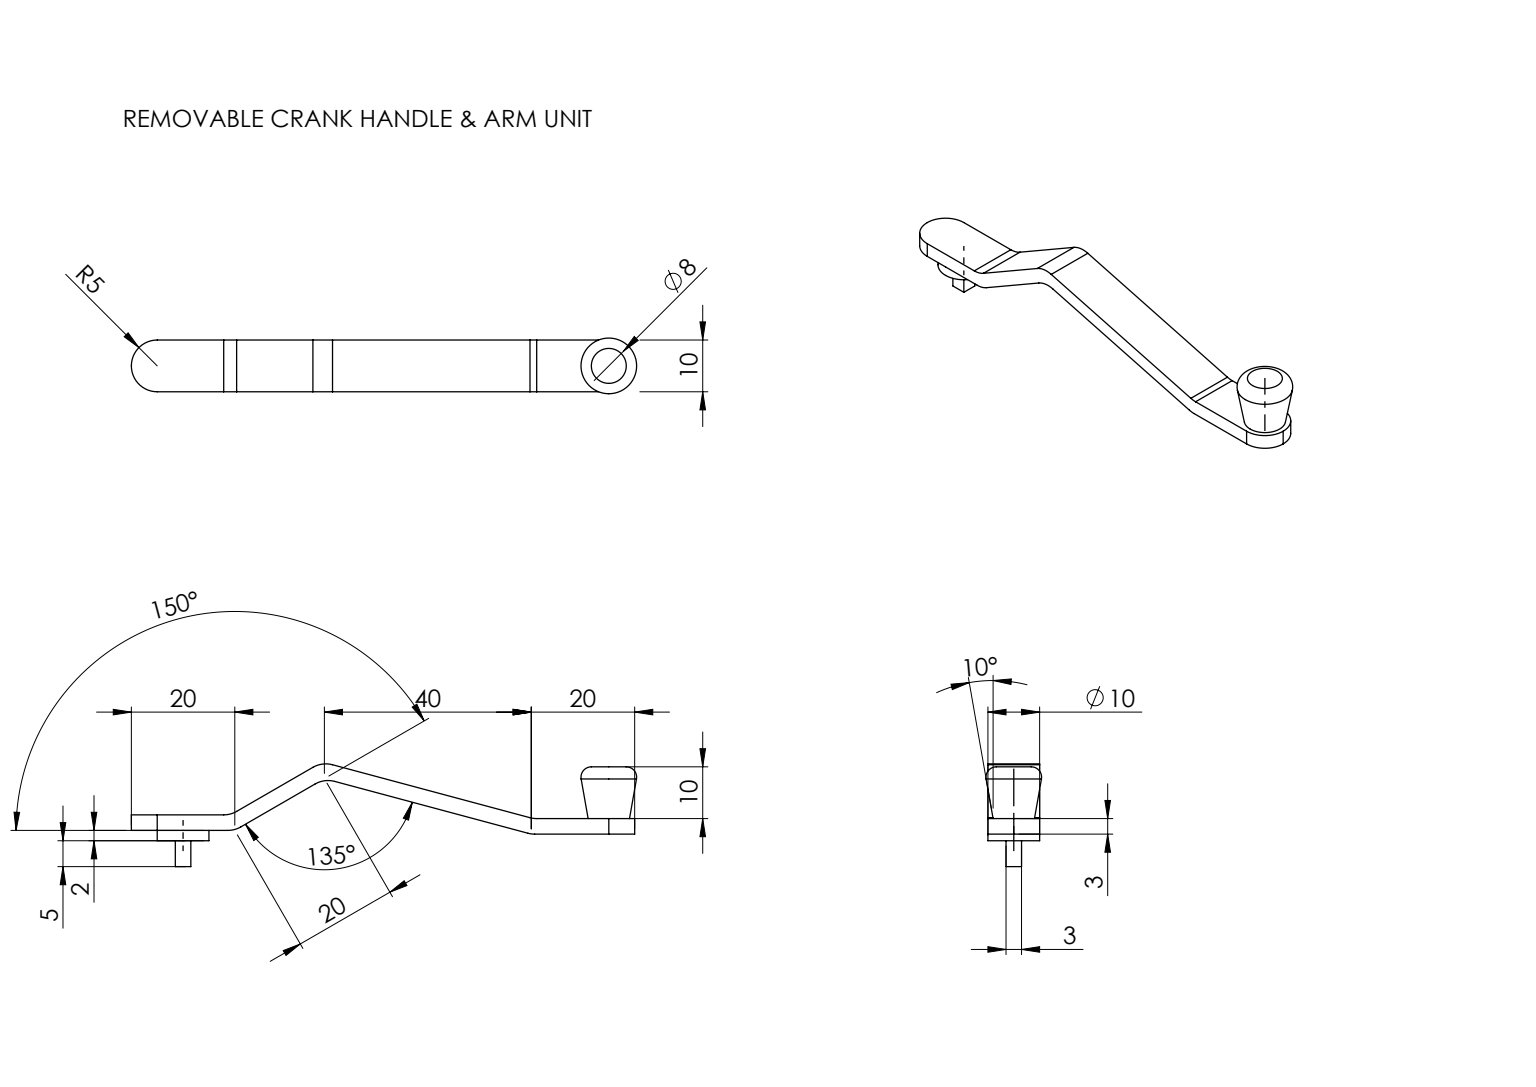
ISO-10303-21;
HEADER;
FILE_DESCRIPTION (('STEP AP214'),
    '1' );
FILE_NAME ('Removable Crank Handle & Arm Unit.step',
    '2026-10-04T07:23:31',
    ( '' ),
    ( '' ),
    'SwSTEP 2.0',
    'SolidWorks 2026',
    '' );
FILE_SCHEMA (( 'AUTOMOTIVE_DESIGN' ));
ENDSEC;

DATA;
#3=ORIENTED_EDGE ( 'NONE', *, *, #5333, .F. ) ;
#12=CARTESIAN_POINT ( 'NONE',  ( 10.00000000000000000, 90.00000000000001421, -5.000000000000000000 ) ) ;
#31=VECTOR ( 'NONE', #278, 1000.000000000000000 ) ;
#33=ORIENTED_EDGE ( 'NONE', *, *, #3191, .T. ) ;
#67=ORIENTED_EDGE ( 'NONE', *, *, #4182, .T. ) ;
#77=ORIENTED_EDGE ( 'NONE', *, *, #7857, .F. ) ;
#83=ORIENTED_EDGE ( 'NONE', *, *, #9025, .F. ) ;
#91=CARTESIAN_POINT ( 'NONE',  ( 1.040834085586084257E-14, 88.00000000000001421, -4.999999999999987566 ) ) ;
#96=SURFACE_SIDE_STYLE ('',( #6842 ) ) ;
#100=LINE ( 'NONE', #5208, #8824 ) ;
#110=DIRECTION ( 'NONE',  ( 0.000000000000000000, 0.000000000000000000, 1.000000000000000000 ) ) ;
#142=ORIENTED_EDGE ( 'NONE', *, *, #10441, .F. ) ;
#177=ADVANCED_FACE ( 'NONE', ( #4290 ), #10361, .F. ) ;
#191=DIRECTION ( 'NONE',  ( 1.000000000000000000, 0.000000000000000000, 0.000000000000000000 ) ) ;
#194=FACE_OUTER_BOUND ( 'NONE', #6105, .T. ) ;
#206=EDGE_LOOP ( 'NONE', ( #9870, #5506, #9937, #2232 ) ) ;
#224=VECTOR ( 'NONE', #10052, 1000.000000000000000 ) ;
#227=CIRCLE ( 'NONE', #6760, 2.000000000000000000 ) ;
#242=ORIENTED_EDGE ( 'NONE', *, *, #1929, .F. ) ;
#243=CIRCLE ( 'NONE', #1136, 3.379762621896238883 ) ;
#250=EDGE_CURVE ( 'NONE', #1860, #1446, #9645, .T. ) ;
#257=VERTEX_POINT ( 'NONE', #2223 ) ;
#259=ORIENTED_EDGE ( 'NONE', *, *, #4096, .F. ) ;
#265=CARTESIAN_POINT ( 'NONE',  ( -1.500000000000000444, 88.00000000000001421, -1.500000000000000222 ) ) ;
#267=DIRECTION ( 'NONE',  ( 0.000000000000000000, 0.000000000000000000, -1.000000000000000000 ) ) ;
#268=EDGE_CURVE ( 'NONE', #2208, #3766, #1396, .T. ) ;
#278=DIRECTION ( 'NONE',  ( -0.000000000000000000, 1.000000000000000000, -0.000000000000000000 ) ) ;
#314=CARTESIAN_POINT ( 'NONE',  ( -5.000000000000000000, 90.00000000000001421, 0.000000000000000000 ) ) ;
#327=CARTESIAN_POINT ( 'NONE',  ( 82.32050807568876394, 92.28203230275514102, 5.000000000000000000 ) ) ;
#347=PRODUCT_DEFINITION_FORMATION_WITH_SPECIFIED_SOURCE ( 'ANY', '', #361, .NOT_KNOWN. ) ;
#361=PRODUCT ( 'Removable Crank Handle & Arm Unit', 'Removable Crank Handle & Arm Unit', '', ( #7853 ) ) ;
#365=DIRECTION ( 'NONE',  ( -0.000000000000000000, -1.000000000000000000, -0.000000000000000000 ) ) ;
#366=ORIENTED_EDGE ( 'NONE', *, *, #7588, .T. ) ;
#367=DIRECTION ( 'NONE',  ( -1.000000000000000000, 5.551115123125781913E-15, 0.000000000000000000 ) ) ;
#371=DIRECTION ( 'NONE',  ( 0.000000000000000000, -0.000000000000000000, 1.000000000000000000 ) ) ;
#377=EDGE_CURVE ( 'NONE', #6765, #3339, #3870, .T. ) ;
#381=DIRECTION ( 'NONE',  ( 0.000000000000000000, 0.000000000000000000, 1.000000000000000000 ) ) ;
#383=ORIENTED_EDGE ( 'NONE', *, *, #5717, .F. ) ;
#385=DIRECTION ( 'NONE',  ( -0.000000000000000000, 1.000000000000000000, -0.000000000000000000 ) ) ;
#387=VERTEX_POINT ( 'NONE', #2812 ) ;
#408=FILL_AREA_STYLE ('',( #5487 ) ) ;
#422=CARTESIAN_POINT ( 'NONE',  ( 1.499999999999999556, 83.00000000000000000, -1.500000000000000222 ) ) ;
#435=DIRECTION ( 'NONE',  ( 0.000000000000000000, 0.000000000000000000, 1.000000000000000000 ) ) ;
#440=LINE ( 'NONE', #3807, #6013 ) ;
#467=ADVANCED_FACE ( 'NONE', ( #4314 ), #3524, .F. ) ;
#470=CARTESIAN_POINT ( 'NONE',  ( -5.000000000000000000, 93.00000000000001421, 0.000000000000000000 ) ) ;
#490=CARTESIAN_POINT ( 'NONE',  ( 1.040834085586084257E-14, 90.00000000000001421, 5.000000000000000000 ) ) ;
#491=CARTESIAN_POINT ( 'NONE',  ( -1.500000000000000444, 88.00000000000001421, 1.499999999999999778 ) ) ;
#505=ORIENTED_EDGE ( 'NONE', *, *, #6617, .F. ) ;
#514=VERTEX_POINT ( 'NONE', #5086 ) ;
#521=CARTESIAN_POINT ( 'NONE',  ( -5.000000000000000000, 93.00000000000001421, 5.000000000000000000 ) ) ;
#529=DIRECTION ( 'NONE',  ( 0.000000000000000000, 0.000000000000000000, -1.000000000000000000 ) ) ;
#533=EDGE_CURVE ( 'NONE', #8829, #4450, #8962, .T. ) ;
#535=CARTESIAN_POINT ( 'NONE',  ( 1.040834085586084257E-14, 90.00000000000001421, 0.000000000000000000 ) ) ;
#544=VERTEX_POINT ( 'NONE', #8636 ) ;
#546=CARTESIAN_POINT ( 'NONE',  ( -1.500000000000000444, 83.00000000000000000, 1.499999999999999778 ) ) ;
#549=ORIENTED_EDGE ( 'NONE', *, *, #6741, .T. ) ;
#564=VERTEX_POINT ( 'NONE', #7642 ) ;
#574=EDGE_CURVE ( 'NONE', #8829, #3039, #9473, .T. ) ;
#587=AXIS2_PLACEMENT_3D ( 'NONE', #4145, #5850, #2623 ) ;
#590=DIRECTION ( 'NONE',  ( -1.000000000000000000, 0.000000000000000000, 0.000000000000000000 ) ) ;
#618=CARTESIAN_POINT ( 'NONE',  ( 8.660254037844401509, 90.00000000000001421, -5.000000000000000000 ) ) ;
#625=ORIENTED_EDGE ( 'NONE', *, *, #3191, .F. ) ;
#648=FACE_OUTER_BOUND ( 'NONE', #8082, .T. ) ;
#653=DIRECTION ( 'NONE',  ( 0.000000000000000000, -0.000000000000000000, 1.000000000000000000 ) ) ;
#658=EDGE_CURVE ( 'NONE', #10864, #2380, #8577, .T. ) ;
#663=CARTESIAN_POINT ( 'NONE',  ( 67.32050807568876394, 89.28203230275514102, 5.000000000000000000 ) ) ;
#672=CIRCLE ( 'NONE', #9503, 2.000000000000000000 ) ;
#677=ORIENTED_EDGE ( 'NONE', *, *, #2132, .T. ) ;
#706=LINE ( 'NONE', #4869, #4614 ) ;
#709=CARTESIAN_POINT ( 'NONE',  ( 67.07963283087528339, 92.45240317130979690, -5.000000000000000000 ) ) ;
#711=EDGE_CURVE ( 'NONE', #8862, #6537, #6673, .T. ) ;
#719=DIRECTION ( 'NONE',  ( -0.000000000000000000, -1.000000000000000000, -0.000000000000000000 ) ) ;
#725=FACE_OUTER_BOUND ( 'NONE', #3287, .T. ) ;
#754=DIRECTION ( 'NONE',  ( 0.000000000000000000, 1.000000000000000000, 0.000000000000000000 ) ) ;
#770=DIRECTION ( 'NONE',  ( 0.000000000000000000, 0.000000000000000000, -1.000000000000000000 ) ) ;
#782=LINE ( 'NONE', #4259, #4639 ) ;
#796=ORIENTED_EDGE ( 'NONE', *, *, #6662, .F. ) ;
#806=VERTEX_POINT ( 'NONE', #6323 ) ;
#810=EDGE_CURVE ( 'NONE', #5184, #1232, #9685, .T. ) ;
#821=FACE_OUTER_BOUND ( 'NONE', #5736, .T. ) ;
#828=DIRECTION ( 'NONE',  ( 0.000000000000000000, -0.000000000000000000, 1.000000000000000000 ) ) ;
#836=FACE_OUTER_BOUND ( 'NONE', #7251, .T. ) ;
#838=CARTESIAN_POINT ( 'NONE',  ( 7.856406460551036197, 93.00000000000001421, -5.000000000000000000 ) ) ;
#839=LINE ( 'NONE', #6642, #10047 ) ;
#862=FACE_OUTER_BOUND ( 'NONE', #9094, .T. ) ;
#875=ORIENTED_EDGE ( 'NONE', *, *, #1882, .T. ) ;
#878=CARTESIAN_POINT ( 'NONE',  ( 8.660254037844401509, 90.00000000000001421, 5.000000000000000000 ) ) ;
#885=VECTOR ( 'NONE', #3233, 1000.000000000000000 ) ;
#894=DIRECTION ( 'NONE',  ( 0.000000000000000000, -0.000000000000000000, 1.000000000000000000 ) ) ;
#898=AXIS2_PLACEMENT_3D ( 'NONE', #9603, #2840, #2892 ) ;
#922=DIRECTION ( 'NONE',  ( -1.000000000000000000, 0.000000000000000000, 0.000000000000000000 ) ) ;
#926=CONICAL_SURFACE ( 'NONE', #3744, 4.000000000000006217, 0.1745329251994333364 ) ;
#934=ORIENTED_EDGE ( 'NONE', *, *, #377, .T. ) ;
#937=CARTESIAN_POINT ( 'NONE',  ( 28.02691073765301155, 94.63433907514509258, 5.000000000000000000 ) ) ;
#944=DIRECTION ( 'NONE',  ( -0.000000000000000000, -0.000000000000000000, 1.000000000000000000 ) ) ;
#955=CARTESIAN_POINT ( 'NONE',  ( 28.89716436598705585, 102.6833647615033840, -5.000000000000000000 ) ) ;
#956=VERTEX_POINT ( 'NONE', #4935 ) ;
#973=FACE_OUTER_BOUND ( 'NONE', #9739, .T. ) ;
#977=ORIENTED_EDGE ( 'NONE', *, *, #1807, .T. ) ;
#1000=CARTESIAN_POINT ( 'NONE',  ( 1.500000000000000000, 83.00000000000000000, 1.500000000000000000 ) ) ;
#1002=ORIENTED_EDGE ( 'NONE', *, *, #1471, .T. ) ;
#1031=DIRECTION ( 'NONE',  ( 0.9659258262890684232, -0.2588190451025202399, 0.000000000000000000 ) ) ;
#1041=DIRECTION ( 'NONE',  ( 0.2588190451025202399, 0.9659258262890684232, -0.000000000000000000 ) ) ;
#1045=CARTESIAN_POINT ( 'NONE',  ( 0.000000000000000000, 83.00000000000000000, 0.000000000000000000 ) ) ;
#1047=AXIS2_PLACEMENT_3D ( 'NONE', #1899, #5280, #4212 ) ;
#1058=ADVANCED_FACE ( 'NONE', ( #4325 ), #4262, .T. ) ;
#1067=PLANE ( 'NONE',  #8873 ) ;
#1072=EDGE_LOOP ( 'NONE', ( #5589, #3090, #10487, #3502 ) ) ;
#1093=ORIENTED_EDGE ( 'NONE', *, *, #10175, .T. ) ;
#1115=CARTESIAN_POINT ( 'NONE',  ( -5.000000000000000000, 90.00000000000001421, 0.000000000000000000 ) ) ;
#1125=VECTOR ( 'NONE', #3487, 1000.000000000000000 ) ;
#1136=AXIS2_PLACEMENT_3D ( 'NONE', #9771, #8895, #5691 ) ;
#1143=ADVANCED_FACE ( 'NONE', ( #648 ), #10756, .F. ) ;
#1160=DIRECTION ( 'NONE',  ( 0.000000000000000000, 0.000000000000000000, 1.000000000000000000 ) ) ;
#1179=CARTESIAN_POINT ( 'NONE',  ( 67.07963283087528339, 92.45240317130979690, 5.000000000000000000 ) ) ;
#1192=DIRECTION ( 'NONE',  ( -0.8660254037844382635, -0.5000000000000004441, 0.000000000000000000 ) ) ;
#1211=EDGE_LOOP ( 'NONE', ( #2757, #9774 ) ) ;
#1216=EDGE_CURVE ( 'NONE', #2617, #9902, #2682, .T. ) ;
#1220=CARTESIAN_POINT ( 'NONE',  ( -1.500000000000000444, 83.00000000000000000, -1.500000000000000222 ) ) ;
#1232=VERTEX_POINT ( 'NONE', #9251 ) ;
#1240=LINE ( 'NONE', #4680, #1791 ) ;
#1249=CIRCLE ( 'NONE', #1405, 5.000000000000000888 ) ;
#1251=DIRECTION ( 'NONE',  ( -0.000000000000000000, -0.000000000000000000, 1.000000000000000000 ) ) ;
#1261=AXIS2_PLACEMENT_3D ( 'NONE', #3295, #5864, #9221 ) ;
#1268=CARTESIAN_POINT ( 'NONE',  ( 28.89716436598705585, 102.6833647615033840, 5.000000000000000000 ) ) ;
#1272=CIRCLE ( 'NONE', #4980, 5.000000000000000000 ) ;
#1281=DIRECTION ( 'NONE',  ( 0.000000000000000000, 0.000000000000000000, 1.000000000000000000 ) ) ;
#1283=VECTOR ( 'NONE', #3007, 1000.000000000000000 ) ;
#1296=CIRCLE ( 'NONE', #10816, 4.999999999999987566 ) ;
#1315=LINE ( 'NONE', #7318, #7623 ) ;
#1316=FACE_OUTER_BOUND ( 'NONE', #4208, .T. ) ;
#1345=EDGE_CURVE ( 'NONE', #8432, #10429, #10558, .T. ) ;
#1351=CARTESIAN_POINT ( 'NONE',  ( 82.32050807568876394, 100.2820323027551268, -3.379762621896238883 ) ) ;
#1371=ORIENTED_EDGE ( 'NONE', *, *, #2509, .F. ) ;
#1372=DIRECTION ( 'NONE',  ( 0.000000000000000000, 1.000000000000000000, 0.000000000000000000 ) ) ;
#1389=LINE ( 'NONE', #1502, #10598 ) ;
#1396=LINE ( 'NONE', #4580, #3474 ) ;
#1405=AXIS2_PLACEMENT_3D ( 'NONE', #5689, #9982, #9871 ) ;
#1410=LINE ( 'NONE', #10588, #10799 ) ;
#1413=AXIS2_PLACEMENT_3D ( 'NONE', #2827, #6168, #5342 ) ;
#1445=ORIENTED_EDGE ( 'NONE', *, *, #3645, .T. ) ;
#1446=VERTEX_POINT ( 'NONE', #8690 ) ;
#1471=EDGE_CURVE ( 'NONE', #3766, #806, #8902, .T. ) ;
#1487=PLANE ( 'NONE',  #3213 ) ;
#1497=EDGE_LOOP ( 'NONE', ( #5465, #8707, #5889, #9627 ) ) ;
#1502=CARTESIAN_POINT ( 'NONE',  ( -10.00000000000000000, 93.00000000000001421, -5.000000000000000000 ) ) ;
#1505=CARTESIAN_POINT ( 'NONE',  ( 82.32050807568876394, 89.28203230275514102, 0.000000000000000000 ) ) ;
#1519=CARTESIAN_POINT ( 'NONE',  ( 11.16025403784440329, 90.66987298107783033, -5.000000000000000000 ) ) ;
#1530=CARTESIAN_POINT ( 'NONE',  ( 10.35640646055103886, 93.66987298107783033, 5.000000000000000000 ) ) ;
#1589=LINE ( 'NONE', #4975, #10478 ) ;
#1593=VECTOR ( 'NONE', #9696, 1000.000000000000000 ) ;
#1601=ORIENTED_EDGE ( 'NONE', *, *, #6187, .F. ) ;
#1610=EDGE_CURVE ( 'NONE', #5184, #10316, #1922, .T. ) ;
#1643=AXIS2_PLACEMENT_3D ( 'NONE', #3566, #4536, #5409 ) ;
#1674=ORIENTED_EDGE ( 'NONE', *, *, #5774, .F. ) ;
#1698=FILL_AREA_STYLE_COLOUR ( '', #4075 ) ;
#1710=ORIENTED_EDGE ( 'NONE', *, *, #3464, .T. ) ;
#1720=VERTEX_POINT ( 'NONE', #91 ) ;
#1733=DIRECTION ( 'NONE',  ( 0.8660254037844382635, 0.5000000000000004441, 0.000000000000000000 ) ) ;
#1745=ORIENTED_EDGE ( 'NONE', *, *, #10441, .T. ) ;
#1769=ORIENTED_EDGE ( 'NONE', *, *, #250, .T. ) ;
#1791=VECTOR ( 'NONE', #7301, 1000.000000000000000 ) ;
#1804=DIRECTION ( 'NONE',  ( 0.000000000000000000, 1.000000000000000000, 0.000000000000000000 ) ) ;
#1807=EDGE_CURVE ( 'NONE', #9105, #9832, #9360, .T. ) ;
#1825=AXIS2_PLACEMENT_3D ( 'NONE', #4036, #4920, #5743 ) ;
#1833=CARTESIAN_POINT ( 'NONE',  ( 82.32050807568876394, 92.28203230275514102, 0.000000000000000000 ) ) ;
#1856=DIRECTION ( 'NONE',  ( 0.8660254037844382635, 0.5000000000000004441, 0.000000000000000000 ) ) ;
#1860=VERTEX_POINT ( 'NONE', #6291 ) ;
#1865=CARTESIAN_POINT ( 'NONE',  ( 27.32050807568876749, 100.0000000000000142, 5.000000000000000000 ) ) ;
#1874=DIRECTION ( 'NONE',  ( -0.000000000000000000, -0.000000000000000000, -1.000000000000000000 ) ) ;
#1882=EDGE_CURVE ( 'NONE', #5496, #4908, #5613, .T. ) ;
#1895=ORIENTED_EDGE ( 'NONE', *, *, #6352, .F. ) ;
#1899=CARTESIAN_POINT ( 'NONE',  ( 1.040834085586084257E-14, 90.00000000000001421, 0.000000000000000000 ) ) ;
#1904=CARTESIAN_POINT ( 'NONE',  ( 0.000000000000000000, 0.000000000000000000, 0.000000000000000000 ) ) ;
#1915=COLOUR_RGB ( '', 0.31764706, 0.68627451, 0.89019608) ;
#1922=LINE ( 'NONE', #7778, #4446 ) ;
#1929=EDGE_CURVE ( 'NONE', #8979, #2617, #2296, .T. ) ;
#1940=ADVANCED_FACE ( 'NONE', ( #194 ), #2768, .T. ) ;
#1959=ORIENTED_EDGE ( 'NONE', *, *, #3062, .T. ) ;
#1976=VERTEX_POINT ( 'NONE', #7979 ) ;
#1988=VERTEX_POINT ( 'NONE', #3554 ) ;
#2078=EDGE_CURVE ( 'NONE', #5999, #5308, #6726, .T. ) ;
#2092=CARTESIAN_POINT ( 'NONE',  ( -1.500000000000000444, 83.00000000000000000, -1.500000000000000222 ) ) ;
#2098=VERTEX_POINT ( 'NONE', #618 ) ;
#2108=SURFACE_STYLE_FILL_AREA ( #408 ) ;
#2116=ORIENTED_EDGE ( 'NONE', *, *, #7733, .T. ) ;
#2123=CARTESIAN_POINT ( 'NONE',  ( 28.02691073765301155, 94.63433907514509258, -5.000000000000000000 ) ) ;
#2130=VERTEX_POINT ( 'NONE', #4835 ) ;
#2132=EDGE_CURVE ( 'NONE', #3067, #8979, #1389, .T. ) ;
#2147=AXIS2_PLACEMENT_3D ( 'NONE', #10891, #3469, #6860 ) ;
#2157=AXIS2_PLACEMENT_3D ( 'NONE', #9612, #3803, #9558 ) ;
#2185=CARTESIAN_POINT ( 'NONE',  ( 1.500000000000000000, 83.00000000000000000, 1.500000000000000000 ) ) ;
#2204=DIRECTION ( 'NONE',  ( -1.000000000000000000, 0.000000000000000000, 0.000000000000000000 ) ) ;
#2205=ORIENTED_EDGE ( 'NONE', *, *, #4118, .F. ) ;
#2208=VERTEX_POINT ( 'NONE', #8230 ) ;
#2215=DIRECTION ( 'NONE',  ( 0.000000000000000000, 0.000000000000000000, 1.000000000000000000 ) ) ;
#2220=ORIENTED_EDGE ( 'NONE', *, *, #9236, .T. ) ;
#2223=CARTESIAN_POINT ( 'NONE',  ( 82.32050807568876394, 102.2820323027551410, 3.379762621896238883 ) ) ;
#2226=DIRECTION ( 'NONE',  ( -1.000000000000000000, -2.775557561562888984E-15, 0.000000000000000000 ) ) ;
#2232=ORIENTED_EDGE ( 'NONE', *, *, #6187, .T. ) ;
#2253=VECTOR ( 'NONE', #8853, 1000.000000000000000 ) ;
#2258=EDGE_CURVE ( 'NONE', #6215, #1976, #839, .T. ) ;
#2267=EDGE_CURVE ( 'NONE', #956, #2130, #6702, .T. ) ;
#2270=CARTESIAN_POINT ( 'NONE',  ( -10.00000000000000000, 90.00000000000001421, 5.000000000000000000 ) ) ;
#2296=CIRCLE ( 'NONE', #9548, 5.000000000000000000 ) ;
#2303=DIRECTION ( 'NONE',  ( 0.000000000000000000, -0.000000000000000000, 1.000000000000000000 ) ) ;
#2348=ORIENTED_EDGE ( 'NONE', *, *, #810, .F. ) ;
#2358=ORIENTED_EDGE ( 'NONE', *, *, #7732, .F. ) ;
#2363=LINE ( 'NONE', #1530, #6371 ) ;
#2366=LINE ( 'NONE', #709, #10099 ) ;
#2380=VERTEX_POINT ( 'NONE', #7463 ) ;
#2383=ORIENTED_EDGE ( 'NONE', *, *, #6366, .F. ) ;
#2388=DIRECTION ( 'NONE',  ( 1.000000000000000000, 0.000000000000000000, 0.000000000000000000 ) ) ;
#2402=ORIENTED_EDGE ( 'NONE', *, *, #250, .F. ) ;
#2430=( GEOMETRIC_REPRESENTATION_CONTEXT ( 3 ) GLOBAL_UNCERTAINTY_ASSIGNED_CONTEXT ( ( #5929 ) ) GLOBAL_UNIT_ASSIGNED_CONTEXT ( ( #9834, #6322, #10564 ) ) REPRESENTATION_CONTEXT ( 'NONE', 'WORKASPACE' ) );
#2437=DIRECTION ( 'NONE',  ( 1.000000000000000000, 0.000000000000000000, 0.000000000000000000 ) ) ;
#2446=VERTEX_POINT ( 'NONE', #9888 ) ;
#2459=AXIS2_PLACEMENT_3D ( 'NONE', #1045, #6129, #371 ) ;
#2465=EDGE_CURVE ( 'NONE', #7827, #3126, #5820, .T. ) ;
#2475=CYLINDRICAL_SURFACE ( 'NONE', #6895, 5.000000000000000000 ) ;
#2478=DIRECTION ( 'NONE',  ( 0.000000000000000000, 0.000000000000000000, 1.000000000000000000 ) ) ;
#2501=CARTESIAN_POINT ( 'NONE',  ( 82.32050807568876394, 92.28203230275514102, 0.000000000000000000 ) ) ;
#2509=EDGE_CURVE ( 'NONE', #1988, #2446, #10184, .T. ) ;
#2535=EDGE_CURVE ( 'NONE', #6001, #1446, #9127, .T. ) ;
#2549=ORIENTED_EDGE ( 'NONE', *, *, #8776, .T. ) ;
#2553=CARTESIAN_POINT ( 'NONE',  ( -5.000000000000000000, 90.00000000000001421, 0.000000000000000000 ) ) ;
#2568=LINE ( 'NONE', #878, #9598 ) ;
#2617=VERTEX_POINT ( 'NONE', #8697 ) ;
#2620=( LENGTH_UNIT ( ) NAMED_UNIT ( * ) SI_UNIT ( .MILLI., .METRE. ) );
#2623=DIRECTION ( 'NONE',  ( 0.000000000000000000, 0.000000000000000000, 1.000000000000000000 ) ) ;
#2635=DIRECTION ( 'NONE',  ( -0.000000000000000000, -0.000000000000000000, 1.000000000000000000 ) ) ;
#2636=ORIENTED_EDGE ( 'NONE', *, *, #7018, .T. ) ;
#2644=ORIENTED_EDGE ( 'NONE', *, *, #7733, .F. ) ;
#2657=CARTESIAN_POINT ( 'NONE',  ( 8.499999999999998224, 92.59807621135333022, 5.000000000000000000 ) ) ;
#2678=VECTOR ( 'NONE', #529, 1000.000000000000000 ) ;
#2682=LINE ( 'NONE', #9149, #3688 ) ;
#2697=CIRCLE ( 'NONE', #3956, 5.000000000000000000 ) ;
#2700=VERTEX_POINT ( 'NONE', #5597 ) ;
#2731=CARTESIAN_POINT ( 'NONE',  ( 68.37372805638788975, 92.28203230275514102, 5.000000000000000000 ) ) ;
#2734=PLANE ( 'NONE',  #2459 ) ;
#2757=ORIENTED_EDGE ( 'NONE', *, *, #7215, .F. ) ;
#2765=FACE_OUTER_BOUND ( 'NONE', #1497, .T. ) ;
#2768=CYLINDRICAL_SURFACE ( 'NONE', #1413, 5.000000000000000000 ) ;
#2771=EDGE_LOOP ( 'NONE', ( #10171, #5911, #8645, #8745 ) ) ;
#2812=CARTESIAN_POINT ( 'NONE',  ( 10.35640646055104064, 93.66987298107783033, 5.000000000000000000 ) ) ;
#2813=ADVANCED_FACE ( 'NONE', ( #7780 ), #2734, .F. ) ;
#2817=VECTOR ( 'NONE', #8387, 1000.000000000000000 ) ;
#2827=CARTESIAN_POINT ( 'NONE',  ( 82.32050807568876394, 0.000000000000000000, 0.000000000000000000 ) ) ;
#2840=DIRECTION ( 'NONE',  ( -0.000000000000000000, -0.000000000000000000, 1.000000000000000000 ) ) ;
#2845=ORIENTED_EDGE ( 'NONE', *, *, #2923, .F. ) ;
#2853=AXIS2_PLACEMENT_3D ( 'NONE', #9859, #5677, #10590 ) ;
#2856=EDGE_CURVE ( 'NONE', #2446, #2130, #5828, .T. ) ;
#2859=CARTESIAN_POINT ( 'NONE',  ( 27.60306914047445304, 97.85373563005803987, 5.000000000000000000 ) ) ;
#2865=CARTESIAN_POINT ( 'NONE',  ( 1.040834085586084257E-14, 88.00000000000001421, 0.000000000000000000 ) ) ;
#2890=FACE_OUTER_BOUND ( 'NONE', #6042, .T. ) ;
#2892=DIRECTION ( 'NONE',  ( -1.000000000000000000, -2.775557561562888984E-15, 0.000000000000000000 ) ) ;
#2905=DIRECTION ( 'NONE',  ( 0.000000000000000000, 0.000000000000000000, -1.000000000000000000 ) ) ;
#2906=DIRECTION ( 'NONE',  ( -1.000000000000000000, 0.000000000000000000, 0.000000000000000000 ) ) ;
#2910=FACE_BOUND ( 'NONE', #7286, .T. ) ;
#2917=ORIENTED_EDGE ( 'NONE', *, *, #9280, .F. ) ;
#2922=PRESENTATION_STYLE_ASSIGNMENT (( #6478 ) ) ;
#2923=EDGE_CURVE ( 'NONE', #9832, #514, #3131, .T. ) ;
#2928=CYLINDRICAL_SURFACE ( 'NONE', #3187, 5.000000000000004441 ) ;
#2934=DIRECTION ( 'NONE',  ( -0.000000000000000000, 1.000000000000000000, -0.000000000000000000 ) ) ;
#2935=AXIS2_PLACEMENT_3D ( 'NONE', #3896, #10686, #2226 ) ;
#2951=DIRECTION ( 'NONE',  ( 0.000000000000000000, 1.000000000000000000, 0.000000000000000000 ) ) ;
#2978=AXIS2_PLACEMENT_3D ( 'NONE', #9100, #6680, #10880 ) ;
#2982=ORIENTED_EDGE ( 'NONE', *, *, #2078, .F. ) ;
#2999=ADVANCED_FACE ( 'NONE', ( #7295 ), #8181, .F. ) ;
#3001=DIRECTION ( 'NONE',  ( 0.000000000000000000, 0.9848077530122080203, 0.1736481776669307198 ) ) ;
#3007=DIRECTION ( 'NONE',  ( 2.126576849575776229E-17, 0.9848077530122080203, -0.1736481776669307198 ) ) ;
#3009=ORIENTED_EDGE ( 'NONE', *, *, #2923, .T. ) ;
#3039=VERTEX_POINT ( 'NONE', #5263 ) ;
#3048=EDGE_CURVE ( 'NONE', #956, #10147, #3155, .T. ) ;
#3058=DIRECTION ( 'NONE',  ( -0.000000000000000000, 0.000000000000000000, -1.000000000000000000 ) ) ;
#3062=EDGE_CURVE ( 'NONE', #10429, #544, #9265, .T. ) ;
#3064=ADVANCED_FACE ( 'NONE', ( #9322 ), #4318, .F. ) ;
#3067=VERTEX_POINT ( 'NONE', #5916 ) ;
#3071=CARTESIAN_POINT ( 'NONE',  ( 66.68467533811312364, 89.45240317130979690, 5.000000000000000000 ) ) ;
#3084=ORIENTED_EDGE ( 'NONE', *, *, #6791, .F. ) ;
#3090=ORIENTED_EDGE ( 'NONE', *, *, #574, .T. ) ;
#3096=CARTESIAN_POINT ( 'NONE',  ( 82.32050807568876394, 99.93473594742127375, -5.349378127920655146 ) ) ;
#3116=ORIENTED_EDGE ( 'NONE', *, *, #9145, .T. ) ;
#3123=CARTESIAN_POINT ( 'NONE',  ( 1.040834085586084257E-14, 90.00000000000001421, -4.999999999999987566 ) ) ;
#3126=VERTEX_POINT ( 'NONE', #3350 ) ;
#3131=LINE ( 'NONE', #663, #885 ) ;
#3143=ORIENTED_EDGE ( 'NONE', *, *, #6741, .F. ) ;
#3155=CIRCLE ( 'NONE', #7238, 5.000000000000000000 ) ;
#3168=DIRECTION ( 'NONE',  ( 0.000000000000000000, 0.000000000000000000, -1.000000000000000000 ) ) ;
#3175=DIRECTION ( 'NONE',  ( 0.000000000000000000, 0.000000000000000000, -1.000000000000000000 ) ) ;
#3184=ORIENTED_EDGE ( 'NONE', *, *, #1345, .T. ) ;
#3185=FACE_OUTER_BOUND ( 'NONE', #6312, .T. ) ;
#3187=AXIS2_PLACEMENT_3D ( 'NONE', #9638, #8803, #5492 ) ;
#3189=CARTESIAN_POINT ( 'NONE',  ( 82.32050807568876394, 102.2820323027551410, 0.000000000000000000 ) ) ;
#3191=EDGE_CURVE ( 'NONE', #2700, #6001, #440, .T. ) ;
#3211=ADVANCED_FACE ( 'NONE', ( #5524 ), #8889, .T. ) ;
#3212=EDGE_LOOP ( 'NONE', ( #9099, #5431, #77, #1769 ) ) ;
#3213=AXIS2_PLACEMENT_3D ( 'NONE', #546, #8113, #4870 ) ;
#3221=ORIENTED_EDGE ( 'NONE', *, *, #4369, .T. ) ;
#3233=DIRECTION ( 'NONE',  ( 1.000000000000000000, 0.000000000000000000, 0.000000000000000000 ) ) ;
#3243=ORIENTED_EDGE ( 'NONE', *, *, #6543, .F. ) ;
#3262=ORIENTED_EDGE ( 'NONE', *, *, #7588, .F. ) ;
#3264=EDGE_LOOP ( 'NONE', ( #7982, #5182, #366, #3243 ) ) ;
#3266=DIRECTION ( 'NONE',  ( 0.000000000000000000, -1.000000000000000000, 0.000000000000000000 ) ) ;
#3272=ADVANCED_FACE ( 'NONE', ( #8781 ), #9617, .F. ) ;
#3284=LINE ( 'NONE', #3123, #6761 ) ;
#3287=EDGE_LOOP ( 'NONE', ( #10439, #7426, #7483, #6618 ) ) ;
#3291=VECTOR ( 'NONE', #10406, 1000.000000000000000 ) ;
#3293=LINE ( 'NONE', #4152, #224 ) ;
#3295=CARTESIAN_POINT ( 'NONE',  ( 0.000000000000000000, 0.000000000000000000, 5.000000000000000000 ) ) ;
#3299=DIRECTION ( 'NONE',  ( 1.000000000000000000, 0.000000000000000000, 0.000000000000000000 ) ) ;
#3302=ORIENTED_EDGE ( 'NONE', *, *, #2465, .F. ) ;
#3307=CARTESIAN_POINT ( 'NONE',  ( 68.37372805638788975, 92.28203230275514102, 5.000000000000000000 ) ) ;
#3322=VECTOR ( 'NONE', #5981, 1000.000000000000000 ) ;
#3323=EDGE_CURVE ( 'NONE', #1232, #8979, #8934, .T. ) ;
#3330=AXIS2_PLACEMENT_3D ( 'NONE', #2859, #2905, #8834 ) ;
#3339=VERTEX_POINT ( 'NONE', #9866 ) ;
#3350=CARTESIAN_POINT ( 'NONE',  ( 25.52691073765301510, 98.96446609406727646, -5.000000000000000000 ) ) ;
#3355=DIRECTION ( 'NONE',  ( 0.000000000000000000, 1.000000000000000000, 0.000000000000000000 ) ) ;
#3361=ORIENTED_EDGE ( 'NONE', *, *, #6141, .T. ) ;
#3365=UNCERTAINTY_MEASURE_WITH_UNIT (LENGTH_MEASURE( 1.000000000000000082E-05 ), #6276, 'distance_accuracy_value', 'NONE');
#3408=ADVANCED_FACE ( 'NONE', ( #821 ), #6019, .F. ) ;
#3412=DIRECTION ( 'NONE',  ( 0.000000000000000000, 0.000000000000000000, 1.000000000000000000 ) ) ;
#3414=CYLINDRICAL_SURFACE ( 'NONE', #7265, 5.000000000000000000 ) ;
#3424=ORIENTED_EDGE ( 'NONE', *, *, #9145, .F. ) ;
#3425=ORIENTED_EDGE ( 'NONE', *, *, #5954, .T. ) ;
#3431=DIRECTION ( 'NONE',  ( 0.000000000000000000, 0.000000000000000000, 1.000000000000000000 ) ) ;
#3434=DIRECTION ( 'NONE',  ( -0.5000000000000005551, 0.8660254037844383745, 0.000000000000000000 ) ) ;
#3440=ORIENTED_EDGE ( 'NONE', *, *, #3323, .F. ) ;
#3447=LINE ( 'NONE', #2731, #3772 ) ;
#3450=ORIENTED_EDGE ( 'NONE', *, *, #6211, .F. ) ;
#3457=MANIFOLD_SOLID_BREP ( 'Boss-Extrude3', #10008 ) ;
#3464=EDGE_CURVE ( 'NONE', #3339, #6001, #6083, .T. ) ;
#3469=DIRECTION ( 'NONE',  ( 0.000000000000000000, -0.000000000000000000, 1.000000000000000000 ) ) ;
#3474=VECTOR ( 'NONE', #7931, 1000.000000000000000 ) ;
#3477=CARTESIAN_POINT ( 'NONE',  ( 66.68467533811312364, 89.45240317130979690, 5.000000000000000000 ) ) ;
#3487=DIRECTION ( 'NONE',  ( -0.000000000000000000, -0.000000000000000000, 1.000000000000000000 ) ) ;
#3502=ORIENTED_EDGE ( 'NONE', *, *, #4369, .F. ) ;
#3521=CIRCLE ( 'NONE', #10432, 5.000000000000000000 ) ;
#3524=PLANE ( 'NONE',  #5279 ) ;
#3554=CARTESIAN_POINT ( 'NONE',  ( 67.97877056362573001, 89.28203230275514102, -5.000000000000000000 ) ) ;
#3556=CARTESIAN_POINT ( 'NONE',  ( 27.32050807568876749, 100.0000000000000142, 5.000000000000000000 ) ) ;
#3566=CARTESIAN_POINT ( 'NONE',  ( 82.32050807568876394, 92.28203230275514102, 0.000000000000000000 ) ) ;
#3583=AXIS2_PLACEMENT_3D ( 'NONE', #314, #3626, #1160 ) ;
#3617=ORIENTED_EDGE ( 'NONE', *, *, #7890, .F. ) ;
#3626=DIRECTION ( 'NONE',  ( -0.000000000000000000, -1.000000000000000000, -0.000000000000000000 ) ) ;
#3643=DIRECTION ( 'NONE',  ( -0.000000000000000000, -1.000000000000000000, -0.000000000000000000 ) ) ;
#3645=EDGE_CURVE ( 'NONE', #2130, #514, #3521, .T. ) ;
#3647=DIRECTION ( 'NONE',  ( 0.000000000000000000, 0.000000000000000000, -1.000000000000000000 ) ) ;
#3669=DIRECTION ( 'NONE',  ( -0.000000000000000000, -0.000000000000000000, 1.000000000000000000 ) ) ;
#3688=VECTOR ( 'NONE', #6792, 1000.000000000000227 ) ;
#3694=DIRECTION ( 'NONE',  ( 0.000000000000000000, 0.000000000000000000, 1.000000000000000000 ) ) ;
#3718=ADVANCED_FACE ( 'NONE', ( #10674 ), #2475, .T. ) ;
#3740=ORIENTED_EDGE ( 'NONE', *, *, #7323, .T. ) ;
#3744=AXIS2_PLACEMENT_3D ( 'NONE', #10225, #6866, #381 ) ;
#3761=CARTESIAN_POINT ( 'NONE',  ( 68.37372805638788975, 97.28203230275514102, 5.000000000000000000 ) ) ;
#3766=VERTEX_POINT ( 'NONE', #9168 ) ;
#3772=VECTOR ( 'NONE', #10198, 1000.000000000000000 ) ;
#3782=SHAPE_REPRESENTATION_RELATIONSHIP ( 'NONE' , 'NONE' ,  #5436, #9554 ) ;
#3788=CIRCLE ( 'NONE', #2853, 5.000000000000000888 ) ;
#3803=DIRECTION ( 'NONE',  ( 0.000000000000000000, 0.000000000000000000, -1.000000000000000000 ) ) ;
#3807=CARTESIAN_POINT ( 'NONE',  ( -1.500000000000000444, 83.00000000000000000, -1.500000000000000222 ) ) ;
#3813=DIRECTION ( 'NONE',  ( 0.000000000000000000, -0.000000000000000000, 1.000000000000000000 ) ) ;
#3816=DIRECTION ( 'NONE',  ( -0.000000000000000000, 1.000000000000000000, -0.000000000000000000 ) ) ;
#3819=ADVANCED_FACE ( 'NONE', ( #3185 ), #5650, .F. ) ;
#3829=CARTESIAN_POINT ( 'NONE',  ( -10.00000000000000000, 93.00000000000001421, 5.000000000000000000 ) ) ;
#3848=AXIS2_PLACEMENT_3D ( 'NONE', #9411, #7700, #7924 ) ;
#3850=ORIENTED_EDGE ( 'NONE', *, *, #4167, .T. ) ;
#3870=LINE ( 'NONE', #7038, #6329 ) ;
#3881=CARTESIAN_POINT ( 'NONE',  ( -10.00000000000000000, 90.00000000000001421, 0.000000000000000000 ) ) ;
#3896=CARTESIAN_POINT ( 'NONE',  ( 68.37372805638788975, 97.28203230275514102, -5.000000000000000000 ) ) ;
#3913=VECTOR ( 'NONE', #8909, 1000.000000000000000 ) ;
#3934=ORIENTED_EDGE ( 'NONE', *, *, #8768, .F. ) ;
#3942=AXIS2_PLACEMENT_3D ( 'NONE', #422, #10838, #8865 ) ;
#3950=ORIENTED_EDGE ( 'NONE', *, *, #5389, .F. ) ;
#3956=AXIS2_PLACEMENT_3D ( 'NONE', #5312, #5260, #3694 ) ;
#3958=DIRECTION ( 'NONE',  ( -0.000000000000000000, -0.000000000000000000, -1.000000000000000000 ) ) ;
#3965=VERTEX_POINT ( 'NONE', #1179 ) ;
#3991=DIRECTION ( 'NONE',  ( 0.000000000000000000, 0.000000000000000000, 1.000000000000000000 ) ) ;
#3997=DIRECTION ( 'NONE',  ( 0.000000000000000000, 1.000000000000000000, 0.000000000000000000 ) ) ;
#4033=CARTESIAN_POINT ( 'NONE',  ( 8.660254037844401509, 95.00000000000001421, -5.000000000000000000 ) ) ;
#4036=CARTESIAN_POINT ( 'NONE',  ( 67.97877056362573001, 94.28203230275514102, -5.000000000000000000 ) ) ;
#4071=CARTESIAN_POINT ( 'NONE',  ( 27.60306914047445304, 97.85373563005803987, -5.000000000000000000 ) ) ;
#4075=COLOUR_RGB ( '', 0.31764706, 0.68627451, 0.89019608) ;
#4085=DIRECTION ( 'NONE',  ( 0.000000000000000000, -0.000000000000000000, 1.000000000000000000 ) ) ;
#4096=EDGE_CURVE ( 'NONE', #2617, #387, #2363, .T. ) ;
#4115=DIRECTION ( 'NONE',  ( -0.000000000000000000, -1.000000000000000000, -0.000000000000000000 ) ) ;
#4118=EDGE_CURVE ( 'NONE', #387, #1232, #5131, .T. ) ;
#4130=DIRECTION ( 'NONE',  ( -1.000000000000000000, 0.000000000000000000, 0.000000000000000000 ) ) ;
#4140=FILL_AREA_STYLE ('',( #1698 ) ) ;
#4145=CARTESIAN_POINT ( 'NONE',  ( 82.32050807568876394, 99.93473594742127375, 0.000000000000000000 ) ) ;
#4152=CARTESIAN_POINT ( 'NONE',  ( 1.499999999999999556, 88.00000000000001421, -1.500000000000000222 ) ) ;
#4156=EDGE_CURVE ( 'NONE', #10414, #2208, #1249, .T. ) ;
#4161=ORIENTED_EDGE ( 'NONE', *, *, #1929, .T. ) ;
#4167=EDGE_CURVE ( 'NONE', #806, #9105, #5790, .T. ) ;
#4172=ORIENTED_EDGE ( 'NONE', *, *, #5717, .T. ) ;
#4175=ADVANCED_FACE ( 'NONE', ( #9816 ), #9151, .T. ) ;
#4182=EDGE_CURVE ( 'NONE', #9832, #1988, #706, .T. ) ;
#4208=EDGE_LOOP ( 'NONE', ( #3302, #8020, #383, #5555, #3221, #677, #4161, #5362, #549, #9118, #8591, #10076, #2549, #1371, #10938, #4939, #5565 ) ) ;
#4212=DIRECTION ( 'NONE',  ( 0.000000000000000000, 0.000000000000000000, 1.000000000000000000 ) ) ;
#4221=CARTESIAN_POINT ( 'NONE',  ( 25.10306914047445659, 102.1838626489802380, -5.000000000000000000 ) ) ;
#4239=AXIS2_PLACEMENT_3D ( 'NONE', #4876, #7397, #5040 ) ;
#4241=EDGE_LOOP ( 'NONE', ( #8135, #6779, #3361, #3184, #3934 ) ) ;
#4259=CARTESIAN_POINT ( 'NONE',  ( 28.89716436598705585, 102.6833647615033840, 5.000000000000000000 ) ) ;
#4262=PLANE ( 'NONE',  #6505 ) ;
#4272=VECTOR ( 'NONE', #3299, 1000.000000000000000 ) ;
#4290=FACE_OUTER_BOUND ( 'NONE', #4241, .T. ) ;
#4293=ORIENTED_EDGE ( 'NONE', *, *, #9215, .T. ) ;
#4301=AXIS2_PLACEMENT_3D ( 'NONE', #5625, #10698, #7320 ) ;
#4303=ORIENTED_EDGE ( 'NONE', *, *, #7096, .T. ) ;
#4305=DIRECTION ( 'NONE',  ( 0.000000000000000000, 0.000000000000000000, 1.000000000000000000 ) ) ;
#4314=FACE_OUTER_BOUND ( 'NONE', #10031, .T. ) ;
#4318=PLANE ( 'NONE',  #4777 ) ;
#4325=FACE_OUTER_BOUND ( 'NONE', #206, .T. ) ;
#4330=ORIENTED_EDGE ( 'NONE', *, *, #1610, .F. ) ;
#4345=DIRECTION ( 'NONE',  ( 0.000000000000000000, -0.000000000000000000, 1.000000000000000000 ) ) ;
#4347=ORIENTED_EDGE ( 'NONE', *, *, #8393, .T. ) ;
#4369=EDGE_CURVE ( 'NONE', #4450, #3067, #100, .T. ) ;
#4379=DIRECTION ( 'NONE',  ( 0.000000000000000000, 0.000000000000000000, 1.000000000000000000 ) ) ;
#4387=ORIENTED_EDGE ( 'NONE', *, *, #810, .T. ) ;
#4394=DIRECTION ( 'NONE',  ( 0.000000000000000000, 1.000000000000000000, 0.000000000000000000 ) ) ;
#4395=MECHANICAL_DESIGN_GEOMETRIC_PRESENTATION_REPRESENTATION('',(#8079),#2430);
#4400=PLANE ( 'NONE',  #7102 ) ;
#4413=DIRECTION ( 'NONE',  ( -0.9659258262890684232, 0.2588190451025202399, 0.000000000000000000 ) ) ;
#4416=DIRECTION ( 'NONE',  ( 0.000000000000000000, -1.000000000000000000, -0.000000000000000000 ) ) ;
#4419=ORIENTED_EDGE ( 'NONE', *, *, #3048, .T. ) ;
#4435=APPLICATION_CONTEXT ( 'automotive_design' ) ;
#4442=DIRECTION ( 'NONE',  ( 0.000000000000000000, 1.000000000000000000, 0.000000000000000000 ) ) ;
#4446=VECTOR ( 'NONE', #4416, 1000.000000000000000 ) ;
#4447=( GEOMETRIC_REPRESENTATION_CONTEXT ( 3 ) GLOBAL_UNCERTAINTY_ASSIGNED_CONTEXT ( ( #7473 ) ) GLOBAL_UNIT_ASSIGNED_CONTEXT ( ( #2620, #8546, #7723 ) ) REPRESENTATION_CONTEXT ( 'NONE', 'WORKASPACE' ) );
#4450=VERTEX_POINT ( 'NONE', #7554 ) ;
#4467=ORIENTED_EDGE ( 'NONE', *, *, #2132, .F. ) ;
#4510=DIRECTION ( 'NONE',  ( 0.000000000000000000, 1.000000000000000000, 0.000000000000000000 ) ) ;
#4528=CARTESIAN_POINT ( 'NONE',  ( 10.00000000000000000, 90.00000000000001421, 5.000000000000000000 ) ) ;
#4536=DIRECTION ( 'NONE',  ( 0.000000000000000000, 1.000000000000000000, 0.000000000000000000 ) ) ;
#4580=CARTESIAN_POINT ( 'NONE',  ( 29.32100596316561081, 99.46396820659043669, -5.000000000000000000 ) ) ;
#4610=FACE_OUTER_BOUND ( 'NONE', #1211, .T. ) ;
#4614=VECTOR ( 'NONE', #4973, 1000.000000000000000 ) ;
#4624=PRODUCT_DEFINITION_CONTEXT ( 'detailed design', #4435, 'design' ) ;
#4633=CARTESIAN_POINT ( 'NONE',  ( 1.500000000000000000, 88.00000000000001421, 1.500000000000000000 ) ) ;
#4637=CIRCLE ( 'NONE', #10794, 3.379762621896238883 ) ;
#4639=VECTOR ( 'NONE', #2635, 1000.000000000000000 ) ;
#4648=DIRECTION ( 'NONE',  ( 1.000000000000000000, 0.000000000000000000, 0.000000000000000000 ) ) ;
#4649=VECTOR ( 'NONE', #8821, 1000.000000000000114 ) ;
#4672=CIRCLE ( 'NONE', #10828, 5.000000000000000000 ) ;
#4673=DIRECTION ( 'NONE',  ( 0.9659258262890684232, -0.2588190451025202399, 0.000000000000000000 ) ) ;
#4680=CARTESIAN_POINT ( 'NONE',  ( 82.32050807568876394, 0.000000000000000000, -5.000000000000000000 ) ) ;
#4713=EDGE_LOOP ( 'NONE', ( #5573, #8193 ) ) ;
#4716=ADVANCED_FACE ( 'NONE', ( #9757 ), #8202, .T. ) ;
#4732=DIRECTION ( 'NONE',  ( 1.000000000000000000, -0.000000000000000000, 1.224646799147353207E-16 ) ) ;
#4748=DIRECTION ( 'NONE',  ( 0.000000000000000000, 1.000000000000000000, 0.000000000000000000 ) ) ;
#4752=ORIENTED_EDGE ( 'NONE', *, *, #268, .T. ) ;
#4771=EDGE_CURVE ( 'NONE', #6537, #8862, #6965, .T. ) ;
#4774=LINE ( 'NONE', #2270, #3913 ) ;
#4777=AXIS2_PLACEMENT_3D ( 'NONE', #7678, #7797, #8616 ) ;
#4827=ORIENTED_EDGE ( 'NONE', *, *, #4771, .F. ) ;
#4835=CARTESIAN_POINT ( 'NONE',  ( 87.32050807568876394, 89.28203230275514102, 0.000000000000000000 ) ) ;
#4836=CIRCLE ( 'NONE', #5201, 4.999999999999987566 ) ;
#4839=ORIENTED_EDGE ( 'NONE', *, *, #10770, .T. ) ;
#4845=EDGE_LOOP ( 'NONE', ( #6814, #2402, #5604, #33 ) ) ;
#4869=CARTESIAN_POINT ( 'NONE',  ( 67.97877056362573001, 89.28203230275514102, 5.000000000000000000 ) ) ;
#4870=DIRECTION ( 'NONE',  ( -1.000000000000000000, 0.000000000000000000, -7.228014483236695816E-17 ) ) ;
#4876=CARTESIAN_POINT ( 'NONE',  ( -1.500000000000000444, 83.00000000000000000, -1.500000000000000222 ) ) ;
#4885=EDGE_LOOP ( 'NONE', ( #1002, #3850, #6301, #4752 ) ) ;
#4907=VECTOR ( 'NONE', #191, 1000.000000000000000 ) ;
#4908=VERTEX_POINT ( 'NONE', #4633 ) ;
#4920=DIRECTION ( 'NONE',  ( 0.000000000000000000, 0.000000000000000000, -1.000000000000000000 ) ) ;
#4923=ORIENTED_EDGE ( 'NONE', *, *, #4156, .F. ) ;
#4935=CARTESIAN_POINT ( 'NONE',  ( 87.32050807568876394, 92.28203230275514102, 0.000000000000000000 ) ) ;
#4937=DIRECTION ( 'NONE',  ( 0.000000000000000000, 0.000000000000000000, -1.000000000000000000 ) ) ;
#4939=ORIENTED_EDGE ( 'NONE', *, *, #1471, .F. ) ;
#4941=DIRECTION ( 'NONE',  ( 0.000000000000000000, 1.000000000000000000, 0.000000000000000000 ) ) ;
#4968=ADVANCED_FACE ( 'NONE', ( #2890 ), #7062, .T. ) ;
#4973=DIRECTION ( 'NONE',  ( -0.000000000000000000, 0.000000000000000000, -1.000000000000000000 ) ) ;
#4975=CARTESIAN_POINT ( 'NONE',  ( 11.16025403784440329, 90.66987298107783033, 5.000000000000000000 ) ) ;
#4976=DIRECTION ( 'NONE',  ( -0.000000000000000000, -1.000000000000000000, -0.000000000000000000 ) ) ;
#4980=AXIS2_PLACEMENT_3D ( 'NONE', #8005, #2951, #435 ) ;
#4992=LINE ( 'NONE', #10785, #4272 ) ;
#5037=EDGE_CURVE ( 'NONE', #3766, #3126, #8887, .T. ) ;
#5038=EDGE_LOOP ( 'NONE', ( #9419, #10879, #3424, #875 ) ) ;
#5040=DIRECTION ( 'NONE',  ( 1.000000000000000000, 0.000000000000000000, 0.000000000000000000 ) ) ;
#5079=SURFACE_STYLE_USAGE ( .BOTH. , #96 ) ;
#5086=CARTESIAN_POINT ( 'NONE',  ( 82.32050807568876394, 89.28203230275514102, 5.000000000000000000 ) ) ;
#5097=DIRECTION ( 'NONE',  ( 1.000000000000000000, 0.000000000000000000, 0.000000000000000000 ) ) ;
#5098=CARTESIAN_POINT ( 'NONE',  ( 87.32050807568876394, 89.28203230275514102, 0.000000000000000000 ) ) ;
#5131=CIRCLE ( 'NONE', #2978, 5.000000000000000000 ) ;
#5158=LINE ( 'NONE', #9399, #6743 ) ;
#5182=ORIENTED_EDGE ( 'NONE', *, *, #9280, .T. ) ;
#5184=VERTEX_POINT ( 'NONE', #521 ) ;
#5185=ORIENTED_EDGE ( 'NONE', *, *, #7857, .T. ) ;
#5186=CIRCLE ( 'NONE', #9920, 5.349378127920655146 ) ;
#5201=AXIS2_PLACEMENT_3D ( 'NONE', #5475, #8839, #1281 ) ;
#5208=CARTESIAN_POINT ( 'NONE',  ( -5.000000000000000000, 0.000000000000000000, -5.000000000000000000 ) ) ;
#5220=CARTESIAN_POINT ( 'NONE',  ( 67.32050807568876394, 92.28203230275514102, 5.000000000000000000 ) ) ;
#5222=DIRECTION ( 'NONE',  ( -0.9659258262890684232, 0.2588190451025202399, 0.000000000000000000 ) ) ;
#5226=VERTEX_POINT ( 'NONE', #3096 ) ;
#5239=LINE ( 'NONE', #4528, #9210 ) ;
#5260=DIRECTION ( 'NONE',  ( 0.000000000000000000, 1.000000000000000000, 0.000000000000000000 ) ) ;
#5263=CARTESIAN_POINT ( 'NONE',  ( -10.00000000000000000, 93.00000000000001421, 0.000000000000000000 ) ) ;
#5279=AXIS2_PLACEMENT_3D ( 'NONE', #7793, #7611, #828 ) ;
#5280=DIRECTION ( 'NONE',  ( 0.000000000000000000, 1.000000000000000000, 0.000000000000000000 ) ) ;
#5308=VERTEX_POINT ( 'NONE', #6036 ) ;
#5312=CARTESIAN_POINT ( 'NONE',  ( 82.32050807568876394, 92.28203230275514102, 0.000000000000000000 ) ) ;
#5333=EDGE_CURVE ( 'NONE', #3965, #1976, #2366, .T. ) ;
#5342=DIRECTION ( 'NONE',  ( 0.000000000000000000, 0.000000000000000000, -1.000000000000000000 ) ) ;
#5345=ORIENTED_EDGE ( 'NONE', *, *, #5954, .F. ) ;
#5347=AXIS2_PLACEMENT_3D ( 'NONE', #6533, #5754, #4937 ) ;
#5357=AXIS2_PLACEMENT_3D ( 'NONE', #5454, #6964, #267 ) ;
#5362=ORIENTED_EDGE ( 'NONE', *, *, #1216, .T. ) ;
#5369=AXIS2_PLACEMENT_3D ( 'NONE', #5220, #8505, #894 ) ;
#5388=ORIENTED_EDGE ( 'NONE', *, *, #4182, .F. ) ;
#5389=EDGE_CURVE ( 'NONE', #8432, #1720, #3284, .T. ) ;
#5405=ORIENTED_EDGE ( 'NONE', *, *, #9013, .F. ) ;
#5408=EDGE_CURVE ( 'NONE', #1988, #806, #8510, .T. ) ;
#5409=DIRECTION ( 'NONE',  ( 0.000000000000000000, 0.000000000000000000, 1.000000000000000000 ) ) ;
#5430=ORIENTED_EDGE ( 'NONE', *, *, #2509, .T. ) ;
#5431=ORIENTED_EDGE ( 'NONE', *, *, #1882, .F. ) ;
#5432=PRODUCT_DEFINITION ( 'UNKNOWN', '', #347, #4624 ) ;
#5436=SHAPE_REPRESENTATION ( 'Removable Crank Handle & Arm Unit', ( #7040 ), #6672 ) ;
#5448=TOROIDAL_SURFACE ( 'NONE', #8248, 3.379762621896238883, 2.000000000000000000 ) ;
#5454=CARTESIAN_POINT ( 'NONE',  ( 1.040834085586084257E-14, 90.00000000000001421, 0.000000000000000000 ) ) ;
#5457=CARTESIAN_POINT ( 'NONE',  ( 28.09696521099633060, 102.8977774788672264, 5.000000000000000000 ) ) ;
#5465=ORIENTED_EDGE ( 'NONE', *, *, #10770, .F. ) ;
#5475=CARTESIAN_POINT ( 'NONE',  ( 1.040834085586084257E-14, 88.00000000000001421, 0.000000000000000000 ) ) ;
#5487=FILL_AREA_STYLE_COLOUR ( '', #1915 ) ;
#5489=MECHANICAL_DESIGN_GEOMETRIC_PRESENTATION_REPRESENTATION('',(#10251),#4447);
#5490=DIRECTION ( 'NONE',  ( 0.000000000000000000, 1.000000000000000000, 0.000000000000000000 ) ) ;
#5492=DIRECTION ( 'NONE',  ( 1.000000000000000000, 0.000000000000000000, 0.000000000000000000 ) ) ;
#5496=VERTEX_POINT ( 'NONE', #1000 ) ;
#5498=FACE_OUTER_BOUND ( 'NONE', #3212, .T. ) ;
#5506=ORIENTED_EDGE ( 'NONE', *, *, #5333, .T. ) ;
#5513=DIRECTION ( 'NONE',  ( 1.000000000000000000, 0.000000000000000000, 0.000000000000000000 ) ) ;
#5524=FACE_OUTER_BOUND ( 'NONE', #8453, .T. ) ;
#5555=ORIENTED_EDGE ( 'NONE', *, *, #6141, .F. ) ;
#5565=ORIENTED_EDGE ( 'NONE', *, *, #5037, .T. ) ;
#5572=CARTESIAN_POINT ( 'NONE',  ( 82.32050807568876394, 92.28203230275514102, -4.000000000000006217 ) ) ;
#5573=ORIENTED_EDGE ( 'NONE', *, *, #9025, .T. ) ;
#5578=CARTESIAN_POINT ( 'NONE',  ( 25.52691073765301510, 98.96446609406727646, 5.000000000000000000 ) ) ;
#5589=ORIENTED_EDGE ( 'NONE', *, *, #533, .F. ) ;
#5597=CARTESIAN_POINT ( 'NONE',  ( -1.500000000000000444, 83.00000000000000000, -1.500000000000000222 ) ) ;
#5604=ORIENTED_EDGE ( 'NONE', *, *, #9215, .F. ) ;
#5613=LINE ( 'NONE', #2185, #1593 ) ;
#5616=ORIENTED_EDGE ( 'NONE', *, *, #658, .F. ) ;
#5625=CARTESIAN_POINT ( 'NONE',  ( -10.00000000000000000, 93.00000000000001421, 5.000000000000000000 ) ) ;
#5633=ADVANCED_FACE ( 'NONE', ( #1316 ), #10593, .T. ) ;
#5650=PLANE ( 'NONE',  #1261 ) ;
#5654=CARTESIAN_POINT ( 'NONE',  ( 8.660254037844401509, 95.00000000000001421, 5.000000000000000000 ) ) ;
#5662=VECTOR ( 'NONE', #4673, 999.9999999999998863 ) ;
#5677=DIRECTION ( 'NONE',  ( -0.000000000000000000, -0.000000000000000000, 1.000000000000000000 ) ) ;
#5689=CARTESIAN_POINT ( 'NONE',  ( 28.02691073765301155, 94.63433907514509258, 5.000000000000000000 ) ) ;
#5691=DIRECTION ( 'NONE',  ( 0.000000000000000000, 0.000000000000000000, 1.000000000000000000 ) ) ;
#5710=DIRECTION ( 'NONE',  ( -1.000000000000000000, 0.000000000000000000, 0.000000000000000000 ) ) ;
#5717=EDGE_CURVE ( 'NONE', #8432, #2098, #7220, .T. ) ;
#5720=AXIS2_PLACEMENT_3D ( 'NONE', #2501, #5898, #9247 ) ;
#5736=EDGE_LOOP ( 'NONE', ( #4923, #6873, #9965, #10173 ) ) ;
#5740=ORIENTED_EDGE ( 'NONE', *, *, #4167, .F. ) ;
#5743=DIRECTION ( 'NONE',  ( -1.000000000000000000, 0.000000000000000000, 0.000000000000000000 ) ) ;
#5754=DIRECTION ( 'NONE',  ( -0.000000000000000000, -1.000000000000000000, -0.000000000000000000 ) ) ;
#5773=CIRCLE ( 'NONE', #2935, 5.000000000000004441 ) ;
#5774=EDGE_CURVE ( 'NONE', #10429, #8432, #6956, .T. ) ;
#5778=CARTESIAN_POINT ( 'NONE',  ( 82.32050807568876394, 92.28203230275514102, 0.000000000000000000 ) ) ;
#5779=CARTESIAN_POINT ( 'NONE',  ( 82.32050807568876394, 102.2820323027551410, -3.379762621896238883 ) ) ;
#5782=ADVANCED_FACE ( 'NONE', ( #7373 ), #8100, .T. ) ;
#5790=LINE ( 'NONE', #3071, #9161 ) ;
#5797=ORIENTED_EDGE ( 'NONE', *, *, #7474, .F. ) ;
#5805=DIRECTION ( 'NONE',  ( 0.000000000000000000, 0.000000000000000000, -1.000000000000000000 ) ) ;
#5820=LINE ( 'NONE', #12, #6712 ) ;
#5828=CIRCLE ( 'NONE', #8990, 5.000000000000000000 ) ;
#5850=DIRECTION ( 'NONE',  ( -0.000000000000000000, -1.000000000000000000, -0.000000000000000000 ) ) ;
#5861=CARTESIAN_POINT ( 'NONE',  ( -10.00000000000000000, 90.00000000000001421, -5.000000000000000000 ) ) ;
#5864=DIRECTION ( 'NONE',  ( 0.000000000000000000, 0.000000000000000000, -1.000000000000000000 ) ) ;
#5889=ORIENTED_EDGE ( 'NONE', *, *, #6791, .T. ) ;
#5898=DIRECTION ( 'NONE',  ( 0.000000000000000000, 1.000000000000000000, 0.000000000000000000 ) ) ;
#5911=ORIENTED_EDGE ( 'NONE', *, *, #4096, .T. ) ;
#5916=CARTESIAN_POINT ( 'NONE',  ( -5.000000000000000000, 93.00000000000001421, -5.000000000000000000 ) ) ;
#5929=UNCERTAINTY_MEASURE_WITH_UNIT (LENGTH_MEASURE( 1.000000000000000082E-05 ), #9834, 'distance_accuracy_value', 'NONE');
#5937=CARTESIAN_POINT ( 'NONE',  ( -1.500000000000000444, 88.00000000000001421, -1.500000000000000222 ) ) ;
#5941=VERTEX_POINT ( 'NONE', #8481 ) ;
#5952=EDGE_LOOP ( 'NONE', ( #4387, #10714, #4467, #4303, #2220 ) ) ;
#5954=EDGE_CURVE ( 'NONE', #564, #10864, #3447, .T. ) ;
#5980=DIRECTION ( 'NONE',  ( -1.000000000000000000, -0.000000000000000000, -7.228014483236695816E-17 ) ) ;
#5981=DIRECTION ( 'NONE',  ( 0.000000000000000000, -1.000000000000000000, 0.000000000000000000 ) ) ;
#5999=VERTEX_POINT ( 'NONE', #7064 ) ;
#6000=ORIENTED_EDGE ( 'NONE', *, *, #2856, .F. ) ;
#6001=VERTEX_POINT ( 'NONE', #265 ) ;
#6006=EDGE_LOOP ( 'NONE', ( #5185, #3116, #4347, #4293 ) ) ;
#6013=VECTOR ( 'NONE', #385, 1000.000000000000000 ) ;
#6019=CYLINDRICAL_SURFACE ( 'NONE', #6200, 4.999999999999997335 ) ;
#6032=LINE ( 'NONE', #5861, #6561 ) ;
#6036=CARTESIAN_POINT ( 'NONE',  ( 11.16025403784440329, 90.66987298107783033, 5.000000000000000000 ) ) ;
#6038=CARTESIAN_POINT ( 'NONE',  ( -1.500000000000000444, 83.00000000000000000, 1.499999999999999778 ) ) ;
#6042=EDGE_LOOP ( 'NONE', ( #9537, #2358, #2644, #6319 ) ) ;
#6055=CARTESIAN_POINT ( 'NONE',  ( 7.856406460551036197, 98.00000000000001421, -5.000000000000000000 ) ) ;
#6063=EDGE_CURVE ( 'NONE', #10316, #8829, #8336, .T. ) ;
#6075=CYLINDRICAL_SURFACE ( 'NONE', #5357, 4.999999999999987566 ) ;
#6083=LINE ( 'NONE', #9441, #6913 ) ;
#6105=EDGE_LOOP ( 'NONE', ( #7706, #10866, #6000, #10603 ) ) ;
#6128=FACE_OUTER_BOUND ( 'NONE', #7508, .T. ) ;
#6129=DIRECTION ( 'NONE',  ( 0.000000000000000000, 1.000000000000000000, 0.000000000000000000 ) ) ;
#6138=ADVANCED_FACE ( 'NONE', ( #8442 ), #3414, .T. ) ;
#6141=EDGE_CURVE ( 'NONE', #4450, #8432, #6032, .T. ) ;
#6143=AXIS2_PLACEMENT_3D ( 'NONE', #3761, #3647, #2906 ) ;
#6155=ADVANCED_FACE ( 'NONE', ( #8389 ), #8340, .F. ) ;
#6168=DIRECTION ( 'NONE',  ( 0.000000000000000000, -1.000000000000000000, 0.000000000000000000 ) ) ;
#6182=ORIENTED_EDGE ( 'NONE', *, *, #2535, .F. ) ;
#6184=VECTOR ( 'NONE', #2388, 1000.000000000000000 ) ;
#6187=EDGE_CURVE ( 'NONE', #6215, #9231, #782, .T. ) ;
#6200=AXIS2_PLACEMENT_3D ( 'NONE', #937, #4305, #10930 ) ;
#6211=EDGE_CURVE ( 'NONE', #1446, #4908, #3293, .T. ) ;
#6215=VERTEX_POINT ( 'NONE', #955 ) ;
#6276=( LENGTH_UNIT ( ) NAMED_UNIT ( * ) SI_UNIT ( .MILLI., .METRE. ) );
#6291=CARTESIAN_POINT ( 'NONE',  ( 1.499999999999999556, 83.00000000000000000, -1.500000000000000222 ) ) ;
#6301=ORIENTED_EDGE ( 'NONE', *, *, #9970, .F. ) ;
#6311=ORIENTED_EDGE ( 'NONE', *, *, #9098, .F. ) ;
#6312=EDGE_LOOP ( 'NONE', ( #7382, #6451, #7884, #7033, #9444, #977, #3009, #2116, #5616, #1745, #796, #8477, #1895, #10730, #2348, #10720, #7216 ) ) ;
#6317=VECTOR ( 'NONE', #2934, 1000.000000000000000 ) ;
#6319=ORIENTED_EDGE ( 'NONE', *, *, #3645, .F. ) ;
#6322=( NAMED_UNIT ( * ) PLANE_ANGLE_UNIT ( ) SI_UNIT ( $, .RADIAN. ) );
#6323=CARTESIAN_POINT ( 'NONE',  ( 66.68467533811312364, 89.45240317130979690, -5.000000000000000000 ) ) ;
#6329=VECTOR ( 'NONE', #3816, 1000.000000000000000 ) ;
#6337=APPLICATION_CONTEXT ( 'automotive_design' ) ;
#6352=EDGE_CURVE ( 'NONE', #387, #5941, #8891, .T. ) ;
#6366=EDGE_CURVE ( 'NONE', #4908, #3339, #9814, .T. ) ;
#6371=VECTOR ( 'NONE', #9929, 1000.000000000000000 ) ;
#6417=CARTESIAN_POINT ( 'NONE',  ( 8.499999999999998224, 92.59807621135333022, 5.000000000000000000 ) ) ;
#6440=CARTESIAN_POINT ( 'NONE',  ( 1.499999999999999556, 83.00000000000000000, -1.500000000000000222 ) ) ;
#6451=ORIENTED_EDGE ( 'NONE', *, *, #2078, .T. ) ;
#6462=DIRECTION ( 'NONE',  ( 0.8660254037844382635, 0.5000000000000004441, 0.000000000000000000 ) ) ;
#6478=SURFACE_STYLE_USAGE ( .BOTH. , #10675 ) ;
#6502=DIRECTION ( 'NONE',  ( 1.445602896647339163E-16, 0.000000000000000000, 1.000000000000000000 ) ) ;
#6505=AXIS2_PLACEMENT_3D ( 'NONE', #7626, #6930, #5222 ) ;
#6511=ORIENTED_EDGE ( 'NONE', *, *, #3464, .F. ) ;
#6518=ORIENTED_EDGE ( 'NONE', *, *, #10713, .F. ) ;
#6528=DIRECTION ( 'NONE',  ( -1.000000000000000000, 0.000000000000000000, 0.000000000000000000 ) ) ;
#6533=CARTESIAN_POINT ( 'NONE',  ( 1.040834085586084257E-14, 90.00000000000001421, 0.000000000000000000 ) ) ;
#6537=VERTEX_POINT ( 'NONE', #9655 ) ;
#6543=EDGE_CURVE ( 'NONE', #6537, #9241, #1410, .T. ) ;
#6561=VECTOR ( 'NONE', #7513, 1000.000000000000000 ) ;
#6573=AXIS2_PLACEMENT_3D ( 'NONE', #1865, #1041, #4413 ) ;
#6582=VECTOR ( 'NONE', #1031, 999.9999999999998863 ) ;
#6587=DIRECTION ( 'NONE',  ( 0.000000000000000000, 0.000000000000000000, 1.000000000000000000 ) ) ;
#6594=DIRECTION ( 'NONE',  ( 0.9659258262890684232, -0.2588190451025202399, 0.000000000000000000 ) ) ;
#6600=DIRECTION ( 'NONE',  ( 0.000000000000000000, 0.000000000000000000, 1.000000000000000000 ) ) ;
#6611=EDGE_LOOP ( 'NONE', ( #2917, #7861, #9607, #2636 ) ) ;
#6617=EDGE_CURVE ( 'NONE', #5941, #9902, #9856, .T. ) ;
#6618=ORIENTED_EDGE ( 'NONE', *, *, #7215, .T. ) ;
#6623=CARTESIAN_POINT ( 'NONE',  ( 82.32050807568876394, 102.2820323027551410, 0.000000000000000000 ) ) ;
#6642=CARTESIAN_POINT ( 'NONE',  ( 28.09696521099633060, 102.8977774788672264, -5.000000000000000000 ) ) ;
#6662=EDGE_CURVE ( 'NONE', #9231, #3965, #7370, .T. ) ;
#6672=( GEOMETRIC_REPRESENTATION_CONTEXT ( 3 ) GLOBAL_UNCERTAINTY_ASSIGNED_CONTEXT ( ( #3365 ) ) GLOBAL_UNIT_ASSIGNED_CONTEXT ( ( #6276, #8074, #8799 ) ) REPRESENTATION_CONTEXT ( 'NONE', 'WORKASPACE' ) );
#6673=CIRCLE ( 'NONE', #9842, 4.000000000000006217 ) ;
#6680=DIRECTION ( 'NONE',  ( 0.000000000000000000, 0.000000000000000000, -1.000000000000000000 ) ) ;
#6702=LINE ( 'NONE', #5098, #3322 ) ;
#6712=VECTOR ( 'NONE', #1733, 1000.000000000000227 ) ;
#6726=CIRCLE ( 'NONE', #9008, 5.000000000000000000 ) ;
#6729=ADVANCED_FACE ( 'NONE', ( #862 ), #8308, .T. ) ;
#6741=EDGE_CURVE ( 'NONE', #9902, #6215, #7629, .T. ) ;
#6743=VECTOR ( 'NONE', #5097, 1000.000000000000000 ) ;
#6760=AXIS2_PLACEMENT_3D ( 'NONE', #7595, #4130, #10140 ) ;
#6761=VECTOR ( 'NONE', #4976, 1000.000000000000000 ) ;
#6765=VERTEX_POINT ( 'NONE', #8251 ) ;
#6779=ORIENTED_EDGE ( 'NONE', *, *, #533, .T. ) ;
#6791=EDGE_CURVE ( 'NONE', #9241, #257, #227, .T. ) ;
#6792=DIRECTION ( 'NONE',  ( 0.8660254037844382635, 0.5000000000000004441, 0.000000000000000000 ) ) ;
#6807=ORIENTED_EDGE ( 'NONE', *, *, #7474, .T. ) ;
#6809=FACE_BOUND ( 'NONE', #9175, .T. ) ;
#6814=ORIENTED_EDGE ( 'NONE', *, *, #2535, .T. ) ;
#6842=SURFACE_STYLE_FILL_AREA ( #4140 ) ;
#6860=DIRECTION ( 'NONE',  ( 1.000000000000000000, 0.000000000000000000, 0.000000000000000000 ) ) ;
#6866=DIRECTION ( 'NONE',  ( 0.000000000000000000, 1.000000000000000000, 0.000000000000000000 ) ) ;
#6873=ORIENTED_EDGE ( 'NONE', *, *, #10175, .F. ) ;
#6891=PRODUCT_DEFINITION_SHAPE ( 'NONE', 'NONE',  #5432 ) ;
#6895=AXIS2_PLACEMENT_3D ( 'NONE', #7346, #5805, #6528 ) ;
#6900=FACE_OUTER_BOUND ( 'NONE', #4885, .T. ) ;
#6913=VECTOR ( 'NONE', #1874, 1000.000000000000000 ) ;
#6930=DIRECTION ( 'NONE',  ( 0.2588190451025202399, 0.9659258262890684232, -0.000000000000000000 ) ) ;
#6955=CIRCLE ( 'NONE', #10475, 5.000000000000000000 ) ;
#6956=CIRCLE ( 'NONE', #7833, 4.999999999999987566 ) ;
#6964=DIRECTION ( 'NONE',  ( -0.000000000000000000, -1.000000000000000000, -0.000000000000000000 ) ) ;
#6965=CIRCLE ( 'NONE', #10820, 4.000000000000006217 ) ;
#7018=EDGE_CURVE ( 'NONE', #9241, #5226, #5186, .T. ) ;
#7033=ORIENTED_EDGE ( 'NONE', *, *, #4156, .T. ) ;
#7038=CARTESIAN_POINT ( 'NONE',  ( -1.500000000000000444, 83.00000000000000000, 1.499999999999999778 ) ) ;
#7040=AXIS2_PLACEMENT_3D ( 'NONE', #1904, #3431, #7048 ) ;
#7048=DIRECTION ( 'NONE',  ( 1.000000000000000000, 0.000000000000000000, 0.000000000000000000 ) ) ;
#7062=CYLINDRICAL_SURFACE ( 'NONE', #1643, 5.000000000000000000 ) ;
#7064=CARTESIAN_POINT ( 'NONE',  ( 8.660254037844401509, 90.00000000000001421, 5.000000000000000000 ) ) ;
#7075=ADVANCED_FACE ( 'NONE', ( #5498 ), #10479, .F. ) ;
#7096=EDGE_CURVE ( 'NONE', #3067, #3039, #6955, .T. ) ;
#7102=AXIS2_PLACEMENT_3D ( 'NONE', #2657, #3434, #1192 ) ;
#7153=ADVANCED_FACE ( 'NONE', ( #6809, #836 ), #10221, .T. ) ;
#7188=ORIENTED_EDGE ( 'NONE', *, *, #1807, .F. ) ;
#7201=FACE_OUTER_BOUND ( 'NONE', #10137, .T. ) ;
#7215=EDGE_CURVE ( 'NONE', #1720, #544, #1296, .T. ) ;
#7216=ORIENTED_EDGE ( 'NONE', *, *, #8768, .T. ) ;
#7220=LINE ( 'NONE', #8049, #10643 ) ;
#7228=EDGE_LOOP ( 'NONE', ( #9074, #10340, #10511, #1093 ) ) ;
#7238=AXIS2_PLACEMENT_3D ( 'NONE', #1833, #10050, #3412 ) ;
#7246=AXIS2_PLACEMENT_3D ( 'NONE', #2092, #7960, #9717 ) ;
#7251=EDGE_LOOP ( 'NONE', ( #5405, #3425, #9325, #10830, #4419 ) ) ;
#7264=ADVANCED_FACE ( 'NONE', ( #4610, #2910 ), #1067, .F. ) ;
#7265=AXIS2_PLACEMENT_3D ( 'NONE', #10216, #4941, #110 ) ;
#7280=DIRECTION ( 'NONE',  ( -1.000000000000000000, -0.000000000000000000, -7.228014483236695816E-17 ) ) ;
#7286=EDGE_LOOP ( 'NONE', ( #3450, #6182, #6511, #2383 ) ) ;
#7295=FACE_OUTER_BOUND ( 'NONE', #4845, .T. ) ;
#7301=DIRECTION ( 'NONE',  ( 0.000000000000000000, -1.000000000000000000, 0.000000000000000000 ) ) ;
#7318=CARTESIAN_POINT ( 'NONE',  ( 1.499999999999999556, 83.00000000000000000, -1.500000000000000222 ) ) ;
#7320=DIRECTION ( 'NONE',  ( 0.000000000000000000, -0.000000000000000000, 1.000000000000000000 ) ) ;
#7323=EDGE_CURVE ( 'NONE', #544, #1720, #4836, .T. ) ;
#7333=FACE_OUTER_BOUND ( 'NONE', #5038, .T. ) ;
#7336=EDGE_CURVE ( 'NONE', #8103, #257, #243, .T. ) ;
#7343=CARTESIAN_POINT ( 'NONE',  ( 82.32050807568876394, 89.28203230275514102, 0.000000000000000000 ) ) ;
#7346=CARTESIAN_POINT ( 'NONE',  ( 8.660254037844401509, 95.00000000000001421, 5.000000000000000000 ) ) ;
#7370=LINE ( 'NONE', #5457, #4649 ) ;
#7373=FACE_OUTER_BOUND ( 'NONE', #5952, .T. ) ;
#7376=ADVANCED_FACE ( 'NONE', ( #7333 ), #1487, .F. ) ;
#7382=ORIENTED_EDGE ( 'NONE', *, *, #9098, .T. ) ;
#7395=EDGE_CURVE ( 'NONE', #7827, #2098, #4672, .T. ) ;
#7397=DIRECTION ( 'NONE',  ( -0.000000000000000000, 0.000000000000000000, 1.000000000000000000 ) ) ;
#7426=ORIENTED_EDGE ( 'NONE', *, *, #1345, .F. ) ;
#7437=AXIS2_PLACEMENT_3D ( 'NONE', #4071, #9245, #922 ) ;
#7463=CARTESIAN_POINT ( 'NONE',  ( 82.32050807568876394, 92.28203230275514102, 5.000000000000000000 ) ) ;
#7472=AXIS2_PLACEMENT_3D ( 'NONE', #2123, #1251, #367 ) ;
#7473=UNCERTAINTY_MEASURE_WITH_UNIT (LENGTH_MEASURE( 1.000000000000000082E-05 ), #2620, 'distance_accuracy_value', 'NONE');
#7474=EDGE_CURVE ( 'NONE', #2098, #5999, #2568, .T. ) ;
#7483=ORIENTED_EDGE ( 'NONE', *, *, #5389, .T. ) ;
#7485=EDGE_LOOP ( 'NONE', ( #1710, #625, #9374, #934 ) ) ;
#7489=DIRECTION ( 'NONE',  ( 0.000000000000000000, 0.000000000000000000, -1.000000000000000000 ) ) ;
#7508=EDGE_LOOP ( 'NONE', ( #1674, #1959, #3740, #3950 ) ) ;
#7513=DIRECTION ( 'NONE',  ( 1.000000000000000000, 0.000000000000000000, 0.000000000000000000 ) ) ;
#7542=DIRECTION ( 'NONE',  ( 0.000000000000000000, 0.000000000000000000, 1.000000000000000000 ) ) ;
#7554=CARTESIAN_POINT ( 'NONE',  ( -5.000000000000000000, 90.00000000000001421, -5.000000000000000000 ) ) ;
#7573=ORIENTED_EDGE ( 'NONE', *, *, #5408, .F. ) ;
#7585=CARTESIAN_POINT ( 'NONE',  ( 67.97877056362573001, 89.28203230275514102, 5.000000000000000000 ) ) ;
#7588=EDGE_CURVE ( 'NONE', #5226, #9241, #8875, .T. ) ;
#7595=CARTESIAN_POINT ( 'NONE',  ( 82.32050807568876394, 100.2820323027551268, 3.379762621896238883 ) ) ;
#7611=DIRECTION ( 'NONE',  ( 0.000000000000000000, 1.000000000000000000, 0.000000000000000000 ) ) ;
#7623=VECTOR ( 'NONE', #6502, 1000.000000000000000 ) ;
#7626=CARTESIAN_POINT ( 'NONE',  ( 28.09696521099633060, 102.8977774788672264, 5.000000000000000000 ) ) ;
#7627=LINE ( 'NONE', #1220, #8852 ) ;
#7629=CIRCLE ( 'NONE', #7437, 5.000000000000000888 ) ;
#7642=CARTESIAN_POINT ( 'NONE',  ( 68.37372805638788975, 92.28203230275514102, -5.000000000000000000 ) ) ;
#7663=EDGE_CURVE ( 'NONE', #5308, #7827, #1589, .T. ) ;
#7678=CARTESIAN_POINT ( 'NONE',  ( 10.00000000000000000, 90.00000000000001421, 5.000000000000000000 ) ) ;
#7700=DIRECTION ( 'NONE',  ( 0.000000000000000000, 1.000000000000000000, 0.000000000000000000 ) ) ;
#7706=ORIENTED_EDGE ( 'NONE', *, *, #3048, .F. ) ;
#7723=( NAMED_UNIT ( * ) SI_UNIT ( $, .STERADIAN. ) SOLID_ANGLE_UNIT ( ) );
#7732=EDGE_CURVE ( 'NONE', #2380, #956, #2697, .T. ) ;
#7733=EDGE_CURVE ( 'NONE', #514, #2380, #8730, .T. ) ;
#7746=CARTESIAN_POINT ( 'NONE',  ( 82.32050807568876394, 99.93473594742127375, 5.349378127920655146 ) ) ;
#7759=CARTESIAN_POINT ( 'NONE',  ( 67.32050807568876394, 92.28203230275514102, 5.000000000000000000 ) ) ;
#7778=CARTESIAN_POINT ( 'NONE',  ( -5.000000000000000000, 90.00000000000001421, 5.000000000000000000 ) ) ;
#7780=FACE_OUTER_BOUND ( 'NONE', #6006, .T. ) ;
#7793=CARTESIAN_POINT ( 'NONE',  ( 67.32050807568876394, 89.28203230275514102, 5.000000000000000000 ) ) ;
#7795=VECTOR ( 'NONE', #3958, 1000.000000000000000 ) ;
#7797=DIRECTION ( 'NONE',  ( -0.5000000000000005551, 0.8660254037844383745, 0.000000000000000000 ) ) ;
#7802=DIRECTION ( 'NONE',  ( 0.000000000000000000, 0.000000000000000000, 1.000000000000000000 ) ) ;
#7825=LINE ( 'NONE', #3556, #6582 ) ;
#7827=VERTEX_POINT ( 'NONE', #1519 ) ;
#7833=AXIS2_PLACEMENT_3D ( 'NONE', #535, #4748, #9974 ) ;
#7853=PRODUCT_CONTEXT ( 'NONE', #6337, 'mechanical' ) ;
#7857=EDGE_CURVE ( 'NONE', #1860, #5496, #1315, .T. ) ;
#7861=ORIENTED_EDGE ( 'NONE', *, *, #711, .T. ) ;
#7864=CARTESIAN_POINT ( 'NONE',  ( 1.040834085586084257E-14, 88.00000000000001421, 0.000000000000000000 ) ) ;
#7884=ORIENTED_EDGE ( 'NONE', *, *, #9976, .T. ) ;
#7890=EDGE_CURVE ( 'NONE', #9231, #5941, #3788, .T. ) ;
#7924=DIRECTION ( 'NONE',  ( 0.000000000000000000, 0.000000000000000000, 1.000000000000000000 ) ) ;
#7931=DIRECTION ( 'NONE',  ( 0.000000000000000000, 0.000000000000000000, -1.000000000000000000 ) ) ;
#7960=DIRECTION ( 'NONE',  ( 1.000000000000000000, 0.000000000000000000, -0.000000000000000000 ) ) ;
#7979=CARTESIAN_POINT ( 'NONE',  ( 67.07963283087528339, 92.45240317130979690, -5.000000000000000000 ) ) ;
#7982=ORIENTED_EDGE ( 'NONE', *, *, #4771, .T. ) ;
#8005=CARTESIAN_POINT ( 'NONE',  ( -5.000000000000000000, 93.00000000000001421, 0.000000000000000000 ) ) ;
#8008=ADVANCED_FACE ( 'NONE', ( #8422 ), #10307, .T. ) ;
#8020=ORIENTED_EDGE ( 'NONE', *, *, #7395, .T. ) ;
#8049=CARTESIAN_POINT ( 'NONE',  ( -10.00000000000000000, 90.00000000000001421, -5.000000000000000000 ) ) ;
#8055=EDGE_LOOP ( 'NONE', ( #2205, #259, #242, #3440 ) ) ;
#8074=( NAMED_UNIT ( * ) PLANE_ANGLE_UNIT ( ) SI_UNIT ( $, .RADIAN. ) );
#8075=CARTESIAN_POINT ( 'NONE',  ( 82.32050807568876394, 92.28203230275514102, 0.000000000000000000 ) ) ;
#8079=STYLED_ITEM ( 'NONE', ( #2922 ), #9554 ) ;
#8082=EDGE_LOOP ( 'NONE', ( #4172, #6807, #6311, #9030 ) ) ;
#8087=DIRECTION ( 'NONE',  ( 0.000000000000000000, 0.000000000000000000, -1.000000000000000000 ) ) ;
#8090=CARTESIAN_POINT ( 'NONE',  ( 1.040834085586084257E-14, 90.00000000000001421, -4.999999999999987566 ) ) ;
#8100=PLANE ( 'NONE',  #4301 ) ;
#8103=VERTEX_POINT ( 'NONE', #5779 ) ;
#8105=AXIS2_PLACEMENT_3D ( 'NONE', #6623, #1372, #653 ) ;
#8113=DIRECTION ( 'NONE',  ( 7.228014483236695816E-17, 0.000000000000000000, -1.000000000000000000 ) ) ;
#8135=ORIENTED_EDGE ( 'NONE', *, *, #6063, .T. ) ;
#8173=DIRECTION ( 'NONE',  ( 0.000000000000000000, 0.000000000000000000, -1.000000000000000000 ) ) ;
#8176=AXIS2_PLACEMENT_3D ( 'NONE', #10649, #3058, #590 ) ;
#8181=PLANE ( 'NONE',  #4239 ) ;
#8193=ORIENTED_EDGE ( 'NONE', *, *, #7336, .T. ) ;
#8202=CYLINDRICAL_SURFACE ( 'NONE', #8176, 5.000000000000004441 ) ;
#8230=CARTESIAN_POINT ( 'NONE',  ( 29.32100596316561081, 99.46396820659043669, 5.000000000000000000 ) ) ;
#8235=AXIS2_PLACEMENT_3D ( 'NONE', #9363, #1804, #4345 ) ;
#8248=AXIS2_PLACEMENT_3D ( 'NONE', #8576, #4394, #10352 ) ;
#8250=AXIS2_PLACEMENT_3D ( 'NONE', #10702, #9095, #2303 ) ;
#8251=CARTESIAN_POINT ( 'NONE',  ( -1.500000000000000444, 83.00000000000000000, 1.499999999999999778 ) ) ;
#8261=ORIENTED_EDGE ( 'NONE', *, *, #2856, .T. ) ;
#8270=ADVANCED_FACE ( 'NONE', ( #6900 ), #10256, .F. ) ;
#8293=VECTOR ( 'NONE', #3168, 1000.000000000000000 ) ;
#8308=CYLINDRICAL_SURFACE ( 'NONE', #9743, 5.000000000000000000 ) ;
#8336=CIRCLE ( 'NONE', #3583, 5.000000000000000000 ) ;
#8340=CYLINDRICAL_SURFACE ( 'NONE', #2147, 4.999999999999999112 ) ;
#8387=DIRECTION ( 'NONE',  ( -0.000000000000000000, -1.000000000000000000, -0.000000000000000000 ) ) ;
#8389=FACE_OUTER_BOUND ( 'NONE', #8055, .T. ) ;
#8393=EDGE_CURVE ( 'NONE', #6765, #2700, #9746, .T. ) ;
#8418=CIRCLE ( 'NONE', #6143, 5.000000000000004441 ) ;
#8422=FACE_OUTER_BOUND ( 'NONE', #3264, .T. ) ;
#8432=VERTEX_POINT ( 'NONE', #8090 ) ;
#8433=DIRECTION ( 'NONE',  ( 0.000000000000000000, 1.000000000000000000, 0.000000000000000000 ) ) ;
#8440=CARTESIAN_POINT ( 'NONE',  ( 1.102066425543451831E-14, 90.00000000000001421, 4.999999999999987566 ) ) ;
#8442=FACE_OUTER_BOUND ( 'NONE', #1072, .T. ) ;
#8448=FACE_OUTER_BOUND ( 'NONE', #6611, .T. ) ;
#8451=VECTOR ( 'NONE', #2437, 1000.000000000000000 ) ;
#8453=EDGE_LOOP ( 'NONE', ( #3617, #1601, #3143, #505 ) ) ;
#8477=ORIENTED_EDGE ( 'NONE', *, *, #7890, .T. ) ;
#8481=CARTESIAN_POINT ( 'NONE',  ( 25.10306914047445659, 102.1838626489802380, 5.000000000000000000 ) ) ;
#8505=DIRECTION ( 'NONE',  ( 0.000000000000000000, 1.000000000000000000, 0.000000000000000000 ) ) ;
#8510=CIRCLE ( 'NONE', #1825, 5.000000000000004441 ) ;
#8546=( NAMED_UNIT ( * ) PLANE_ANGLE_UNIT ( ) SI_UNIT ( $, .RADIAN. ) );
#8566=LINE ( 'NONE', #6038, #9570 ) ;
#8573=CARTESIAN_POINT ( 'NONE',  ( 25.52691073765301510, 98.96446609406727646, 5.000000000000000000 ) ) ;
#8576=CARTESIAN_POINT ( 'NONE',  ( 82.32050807568876394, 100.2820323027551268, 0.000000000000000000 ) ) ;
#8577=LINE ( 'NONE', #7759, #4907 ) ;
#8591=ORIENTED_EDGE ( 'NONE', *, *, #10713, .T. ) ;
#8616=DIRECTION ( 'NONE',  ( -0.8660254037844382635, -0.5000000000000004441, 0.000000000000000000 ) ) ;
#8630=LINE ( 'NONE', #8573, #1125 ) ;
#8634=ADVANCED_FACE ( 'NONE', ( #10243 ), #4400, .T. ) ;
#8636=CARTESIAN_POINT ( 'NONE',  ( 1.102066425543451831E-14, 88.00000000000001421, 4.999999999999987566 ) ) ;
#8645=ORIENTED_EDGE ( 'NONE', *, *, #6352, .T. ) ;
#8690=CARTESIAN_POINT ( 'NONE',  ( 1.499999999999999556, 88.00000000000001421, -1.500000000000000222 ) ) ;
#8697=CARTESIAN_POINT ( 'NONE',  ( 10.35640646055104064, 93.66987298107783033, -5.000000000000000000 ) ) ;
#8707=ORIENTED_EDGE ( 'NONE', *, *, #7018, .F. ) ;
#8730=LINE ( 'NONE', #327, #31 ) ;
#8745=ORIENTED_EDGE ( 'NONE', *, *, #6617, .T. ) ;
#8768=EDGE_CURVE ( 'NONE', #10316, #10429, #4774, .T. ) ;
#8776=EDGE_CURVE ( 'NONE', #10147, #2446, #1240, .T. ) ;
#8781=FACE_OUTER_BOUND ( 'NONE', #7485, .T. ) ;
#8799=( NAMED_UNIT ( * ) SI_UNIT ( $, .STERADIAN. ) SOLID_ANGLE_UNIT ( ) );
#8803=DIRECTION ( 'NONE',  ( 0.000000000000000000, -0.000000000000000000, 1.000000000000000000 ) ) ;
#8821=DIRECTION ( 'NONE',  ( 0.9659258262890684232, -0.2588190451025202399, 0.000000000000000000 ) ) ;
#8824=VECTOR ( 'NONE', #8433, 1000.000000000000000 ) ;
#8829=VERTEX_POINT ( 'NONE', #3881 ) ;
#8834=DIRECTION ( 'NONE',  ( -1.000000000000000000, 0.000000000000000000, 0.000000000000000000 ) ) ;
#8839=DIRECTION ( 'NONE',  ( 0.000000000000000000, 1.000000000000000000, 0.000000000000000000 ) ) ;
#8846=CARTESIAN_POINT ( 'NONE',  ( 27.32050807568876749, 100.0000000000000142, -5.000000000000000000 ) ) ;
#8852=VECTOR ( 'NONE', #4648, 1000.000000000000000 ) ;
#8853=DIRECTION ( 'NONE',  ( 1.000000000000000000, 0.000000000000000000, 0.000000000000000000 ) ) ;
#8856=DIRECTION ( 'NONE',  ( 1.000000000000000000, 0.000000000000000000, 0.000000000000000000 ) ) ;
#8862=VERTEX_POINT ( 'NONE', #10519 ) ;
#8865=DIRECTION ( 'NONE',  ( 1.445602896647339163E-16, 0.000000000000000000, 1.000000000000000000 ) ) ;
#8873=AXIS2_PLACEMENT_3D ( 'NONE', #2865, #4442, #3813 ) ;
#8875=CIRCLE ( 'NONE', #587, 5.349378127920655146 ) ;
#8887=CIRCLE ( 'NONE', #7472, 5.000000000000000888 ) ;
#8889=CYLINDRICAL_SURFACE ( 'NONE', #3330, 5.000000000000000888 ) ;
#8891=LINE ( 'NONE', #6417, #9737 ) ;
#8895=DIRECTION ( 'NONE',  ( 0.000000000000000000, 1.000000000000000000, 0.000000000000000000 ) ) ;
#8902=LINE ( 'NONE', #8846, #5662 ) ;
#8909=DIRECTION ( 'NONE',  ( 1.000000000000000000, 0.000000000000000000, 0.000000000000000000 ) ) ;
#8911=ADVANCED_FACE ( 'NONE', ( #7201 ), #2928, .F. ) ;
#8934=LINE ( 'NONE', #10757, #8293 ) ;
#8961=TOROIDAL_SURFACE ( 'NONE', #3848, 3.379762621896238883, 2.000000000000000000 ) ;
#8962=CIRCLE ( 'NONE', #10194, 5.000000000000000000 ) ;
#8979=VERTEX_POINT ( 'NONE', #838 ) ;
#8990=AXIS2_PLACEMENT_3D ( 'NONE', #7343, #719, #3991 ) ;
#9008=AXIS2_PLACEMENT_3D ( 'NONE', #5654, #10726, #5710 ) ;
#9013=EDGE_CURVE ( 'NONE', #564, #10147, #4992, .T. ) ;
#9025=EDGE_CURVE ( 'NONE', #257, #8103, #4637, .T. ) ;
#9030=ORIENTED_EDGE ( 'NONE', *, *, #5774, .T. ) ;
#9074=ORIENTED_EDGE ( 'NONE', *, *, #9976, .F. ) ;
#9079=ADVANCED_FACE ( 'NONE', ( #725 ), #10725, .T. ) ;
#9094=EDGE_LOOP ( 'NONE', ( #10124, #9438, #4330, #9968 ) ) ;
#9095=DIRECTION ( 'NONE',  ( 0.000000000000000000, 1.000000000000000000, 0.000000000000000000 ) ) ;
#9098=EDGE_CURVE ( 'NONE', #10429, #5999, #5158, .T. ) ;
#9099=ORIENTED_EDGE ( 'NONE', *, *, #6211, .T. ) ;
#9100=CARTESIAN_POINT ( 'NONE',  ( 7.856406460551036197, 98.00000000000001421, 5.000000000000000000 ) ) ;
#9105=VERTEX_POINT ( 'NONE', #3477 ) ;
#9118=ORIENTED_EDGE ( 'NONE', *, *, #2258, .T. ) ;
#9127=LINE ( 'NONE', #5937, #8451 ) ;
#9145=EDGE_CURVE ( 'NONE', #5496, #6765, #8566, .T. ) ;
#9147=ADVANCED_FACE ( 'NONE', ( #8448 ), #926, .T. ) ;
#9149=CARTESIAN_POINT ( 'NONE',  ( 8.499999999999998224, 92.59807621135333022, -5.000000000000000000 ) ) ;
#9151=PLANE ( 'NONE',  #8105 ) ;
#9161=VECTOR ( 'NONE', #4085, 1000.000000000000000 ) ;
#9168=CARTESIAN_POINT ( 'NONE',  ( 29.32100596316561081, 99.46396820659043669, -5.000000000000000000 ) ) ;
#9175=EDGE_LOOP ( 'NONE', ( #4827, #9844 ) ) ;
#9190=EDGE_LOOP ( 'NONE', ( #2982, #5797, #9250, #10731 ) ) ;
#9210=VECTOR ( 'NONE', #1856, 1000.000000000000227 ) ;
#9215=EDGE_CURVE ( 'NONE', #2700, #1860, #7627, .T. ) ;
#9221=DIRECTION ( 'NONE',  ( -1.000000000000000000, 0.000000000000000000, -0.000000000000000000 ) ) ;
#9231=VERTEX_POINT ( 'NONE', #1268 ) ;
#9236=EDGE_CURVE ( 'NONE', #3039, #5184, #1272, .T. ) ;
#9241=VERTEX_POINT ( 'NONE', #7746 ) ;
#9245=DIRECTION ( 'NONE',  ( 0.000000000000000000, 0.000000000000000000, -1.000000000000000000 ) ) ;
#9247=DIRECTION ( 'NONE',  ( 0.000000000000000000, 0.000000000000000000, 1.000000000000000000 ) ) ;
#9250=ORIENTED_EDGE ( 'NONE', *, *, #7395, .F. ) ;
#9251=CARTESIAN_POINT ( 'NONE',  ( 7.856406460551036197, 93.00000000000001421, 5.000000000000000000 ) ) ;
#9265=LINE ( 'NONE', #8440, #2817 ) ;
#9280=EDGE_CURVE ( 'NONE', #8862, #5226, #10652, .T. ) ;
#9322=FACE_OUTER_BOUND ( 'NONE', #7228, .T. ) ;
#9325=ORIENTED_EDGE ( 'NONE', *, *, #658, .T. ) ;
#9360=CIRCLE ( 'NONE', #898, 5.000000000000004441 ) ;
#9363=CARTESIAN_POINT ( 'NONE',  ( -10.00000000000000000, 90.00000000000001421, 5.000000000000000000 ) ) ;
#9374=ORIENTED_EDGE ( 'NONE', *, *, #8393, .F. ) ;
#9390=CARTESIAN_POINT ( 'NONE',  ( -5.000000000000000000, 90.00000000000001421, 5.000000000000000000 ) ) ;
#9399=CARTESIAN_POINT ( 'NONE',  ( -10.00000000000000000, 90.00000000000001421, 5.000000000000000000 ) ) ;
#9411=CARTESIAN_POINT ( 'NONE',  ( 82.32050807568876394, 100.2820323027551268, 0.000000000000000000 ) ) ;
#9416=DIRECTION ( 'NONE',  ( -1.000000000000000000, 0.000000000000000000, 0.000000000000000000 ) ) ;
#9419=ORIENTED_EDGE ( 'NONE', *, *, #6366, .T. ) ;
#9438=ORIENTED_EDGE ( 'NONE', *, *, #6063, .F. ) ;
#9441=CARTESIAN_POINT ( 'NONE',  ( -1.500000000000000444, 88.00000000000001421, -1.500000000000000222 ) ) ;
#9444=ORIENTED_EDGE ( 'NONE', *, *, #9970, .T. ) ;
#9469=CARTESIAN_POINT ( 'NONE',  ( 82.32050807568876394, 92.28203230275514102, -5.000000000000000000 ) ) ;
#9473=LINE ( 'NONE', #9529, #3291 ) ;
#9503=AXIS2_PLACEMENT_3D ( 'NONE', #1351, #4732, #8087 ) ;
#9529=CARTESIAN_POINT ( 'NONE',  ( -10.00000000000000000, 93.00000000000001421, 0.000000000000000000 ) ) ;
#9537=ORIENTED_EDGE ( 'NONE', *, *, #2267, .F. ) ;
#9548=AXIS2_PLACEMENT_3D ( 'NONE', #6055, #3669, #9416 ) ;
#9554=ADVANCED_BREP_SHAPE_REPRESENTATION ( '', ( #3457, #7040 ), #6672 ) ;
#9558=DIRECTION ( 'NONE',  ( -1.000000000000000000, 0.000000000000000000, -0.000000000000000000 ) ) ;
#9570=VECTOR ( 'NONE', #5980, 1000.000000000000000 ) ;
#9584=DIRECTION ( 'NONE',  ( 0.000000000000000000, 0.000000000000000000, 1.000000000000000000 ) ) ;
#9598=VECTOR ( 'NONE', #944, 1000.000000000000000 ) ;
#9603=CARTESIAN_POINT ( 'NONE',  ( 67.97877056362573001, 94.28203230275514102, 5.000000000000000000 ) ) ;
#9607=ORIENTED_EDGE ( 'NONE', *, *, #6543, .T. ) ;
#9612=CARTESIAN_POINT ( 'NONE',  ( 0.000000000000000000, 0.000000000000000000, -5.000000000000000000 ) ) ;
#9617=PLANE ( 'NONE',  #7246 ) ;
#9627=ORIENTED_EDGE ( 'NONE', *, *, #7336, .F. ) ;
#9638=CARTESIAN_POINT ( 'NONE',  ( 68.37372805638788975, 97.28203230275514102, 5.000000000000000000 ) ) ;
#9645=LINE ( 'NONE', #6440, #6317 ) ;
#9647=ADVANCED_FACE ( 'NONE', ( #6128 ), #6075, .T. ) ;
#9655=CARTESIAN_POINT ( 'NONE',  ( 82.32050807568876394, 92.28203230275514102, 4.000000000000006217 ) ) ;
#9685=LINE ( 'NONE', #3829, #2253 ) ;
#9696=DIRECTION ( 'NONE',  ( -0.000000000000000000, 1.000000000000000000, -0.000000000000000000 ) ) ;
#9704=CARTESIAN_POINT ( 'NONE',  ( 25.10306914047445659, 102.1838626489802380, 5.000000000000000000 ) ) ;
#9717=DIRECTION ( 'NONE',  ( -0.000000000000000000, 0.000000000000000000, -1.000000000000000000 ) ) ;
#9737=VECTOR ( 'NONE', #6462, 1000.000000000000227 ) ;
#9739=EDGE_LOOP ( 'NONE', ( #3262, #4839, #83, #3084 ) ) ;
#9743=AXIS2_PLACEMENT_3D ( 'NONE', #2553, #3266, #7489 ) ;
#9746=LINE ( 'NONE', #10635, #7795 ) ;
#9757=FACE_OUTER_BOUND ( 'NONE', #9791, .T. ) ;
#9771=CARTESIAN_POINT ( 'NONE',  ( 82.32050807568876394, 102.2820323027551410, 0.000000000000000000 ) ) ;
#9774=ORIENTED_EDGE ( 'NONE', *, *, #7323, .F. ) ;
#9791=EDGE_LOOP ( 'NONE', ( #7188, #5740, #7573, #5388 ) ) ;
#9814=LINE ( 'NONE', #491, #10456 ) ;
#9816=FACE_OUTER_BOUND ( 'NONE', #4713, .T. ) ;
#9832=VERTEX_POINT ( 'NONE', #7585 ) ;
#9834=( LENGTH_UNIT ( ) NAMED_UNIT ( * ) SI_UNIT ( .MILLI., .METRE. ) );
#9842=AXIS2_PLACEMENT_3D ( 'NONE', #8075, #5490, #2215 ) ;
#9844=ORIENTED_EDGE ( 'NONE', *, *, #711, .F. ) ;
#9856=LINE ( 'NONE', #9704, #2678 ) ;
#9859=CARTESIAN_POINT ( 'NONE',  ( 27.60306914047445304, 97.85373563005803987, 5.000000000000000000 ) ) ;
#9866=CARTESIAN_POINT ( 'NONE',  ( -1.500000000000000444, 88.00000000000001421, 1.499999999999999778 ) ) ;
#9870=ORIENTED_EDGE ( 'NONE', *, *, #6662, .T. ) ;
#9871=DIRECTION ( 'NONE',  ( -1.000000000000000000, 0.000000000000000000, 0.000000000000000000 ) ) ;
#9888=CARTESIAN_POINT ( 'NONE',  ( 82.32050807568876394, 89.28203230275514102, -5.000000000000000000 ) ) ;
#9902=VERTEX_POINT ( 'NONE', #4221 ) ;
#9920=AXIS2_PLACEMENT_3D ( 'NONE', #10526, #365, #6587 ) ;
#9929=DIRECTION ( 'NONE',  ( -0.000000000000000000, -0.000000000000000000, 1.000000000000000000 ) ) ;
#9937=ORIENTED_EDGE ( 'NONE', *, *, #2258, .F. ) ;
#9965=ORIENTED_EDGE ( 'NONE', *, *, #5037, .F. ) ;
#9968=ORIENTED_EDGE ( 'NONE', *, *, #9236, .F. ) ;
#9970=EDGE_CURVE ( 'NONE', #2208, #9105, #7825, .T. ) ;
#9974=DIRECTION ( 'NONE',  ( 0.000000000000000000, 0.000000000000000000, 1.000000000000000000 ) ) ;
#9976=EDGE_CURVE ( 'NONE', #5308, #10414, #5239, .T. ) ;
#9982=DIRECTION ( 'NONE',  ( 0.000000000000000000, 0.000000000000000000, -1.000000000000000000 ) ) ;
#10008=CLOSED_SHELL ( 'NONE', ( #10936, #8008, #9647, #7264, #9079, #1143, #467, #7153, #1058, #8634, #5782, #177, #3064, #8270, #3819, #5633, #3718, #6155, #8911, #4716, #3408, #3211, #4968, #1940, #6729, #6138, #9147, #4175, #10920, #7075, #7376, #3272, #2999, #2813 ) ) ;
#10031=EDGE_LOOP ( 'NONE', ( #2845, #67, #5430, #8261, #1445 ) ) ;
#10047=VECTOR ( 'NONE', #6594, 1000.000000000000114 ) ;
#10050=DIRECTION ( 'NONE',  ( 0.000000000000000000, 1.000000000000000000, 0.000000000000000000 ) ) ;
#10052=DIRECTION ( 'NONE',  ( 1.445602896647339163E-16, 0.000000000000000000, 1.000000000000000000 ) ) ;
#10076=ORIENTED_EDGE ( 'NONE', *, *, #9013, .T. ) ;
#10099=VECTOR ( 'NONE', #3175, 1000.000000000000000 ) ;
#10124=ORIENTED_EDGE ( 'NONE', *, *, #574, .F. ) ;
#10132=CARTESIAN_POINT ( 'NONE',  ( 67.32050807568876394, 89.28203230275514102, -5.000000000000000000 ) ) ;
#10137=EDGE_LOOP ( 'NONE', ( #142, #5345, #6518, #3 ) ) ;
#10140=DIRECTION ( 'NONE',  ( 0.000000000000000000, 0.000000000000000000, 1.000000000000000000 ) ) ;
#10147=VERTEX_POINT ( 'NONE', #9469 ) ;
#10171=ORIENTED_EDGE ( 'NONE', *, *, #1216, .F. ) ;
#10173=ORIENTED_EDGE ( 'NONE', *, *, #268, .F. ) ;
#10175=EDGE_CURVE ( 'NONE', #3126, #10414, #8630, .T. ) ;
#10184=LINE ( 'NONE', #10132, #6184 ) ;
#10194=AXIS2_PLACEMENT_3D ( 'NONE', #1115, #3643, #9584 ) ;
#10198=DIRECTION ( 'NONE',  ( -0.000000000000000000, -0.000000000000000000, 1.000000000000000000 ) ) ;
#10205=PRESENTATION_STYLE_ASSIGNMENT (( #5079 ) ) ;
#10216=CARTESIAN_POINT ( 'NONE',  ( -5.000000000000000000, 0.000000000000000000, 0.000000000000000000 ) ) ;
#10221=PLANE ( 'NONE',  #5369 ) ;
#10225=CARTESIAN_POINT ( 'NONE',  ( 82.32050807568876394, 92.28203230275514102, 0.000000000000000000 ) ) ;
#10243=FACE_OUTER_BOUND ( 'NONE', #2771, .T. ) ;
#10251=STYLED_ITEM ( 'NONE', ( #10205 ), #3457 ) ;
#10256=PLANE ( 'NONE',  #6573 ) ;
#10269=SHAPE_DEFINITION_REPRESENTATION ( #6891, #5436 ) ;
#10307=CONICAL_SURFACE ( 'NONE', #5720, 4.000000000000006217, 0.1745329251994333364 ) ;
#10316=VERTEX_POINT ( 'NONE', #9390 ) ;
#10340=ORIENTED_EDGE ( 'NONE', *, *, #7663, .T. ) ;
#10352=DIRECTION ( 'NONE',  ( 0.000000000000000000, 0.000000000000000000, 1.000000000000000000 ) ) ;
#10361=PLANE ( 'NONE',  #8235 ) ;
#10406=DIRECTION ( 'NONE',  ( 0.000000000000000000, 1.000000000000000000, 0.000000000000000000 ) ) ;
#10414=VERTEX_POINT ( 'NONE', #5578 ) ;
#10429=VERTEX_POINT ( 'NONE', #490 ) ;
#10432=AXIS2_PLACEMENT_3D ( 'NONE', #1505, #4115, #6600 ) ;
#10439=ORIENTED_EDGE ( 'NONE', *, *, #3062, .F. ) ;
#10441=EDGE_CURVE ( 'NONE', #10864, #3965, #8418, .T. ) ;
#10456=VECTOR ( 'NONE', #7280, 1000.000000000000000 ) ;
#10475=AXIS2_PLACEMENT_3D ( 'NONE', #470, #3355, #4379 ) ;
#10478=VECTOR ( 'NONE', #770, 1000.000000000000000 ) ;
#10479=PLANE ( 'NONE',  #3942 ) ;
#10487=ORIENTED_EDGE ( 'NONE', *, *, #7096, .F. ) ;
#10511=ORIENTED_EDGE ( 'NONE', *, *, #2465, .T. ) ;
#10519=CARTESIAN_POINT ( 'NONE',  ( 82.32050807568876394, 92.28203230275514102, -4.000000000000006217 ) ) ;
#10526=CARTESIAN_POINT ( 'NONE',  ( 82.32050807568876394, 99.93473594742127375, 0.000000000000000000 ) ) ;
#10558=CIRCLE ( 'NONE', #1047, 4.999999999999987566 ) ;
#10564=( NAMED_UNIT ( * ) SI_UNIT ( $, .STERADIAN. ) SOLID_ANGLE_UNIT ( ) );
#10588=CARTESIAN_POINT ( 'NONE',  ( 82.32050807568876394, 92.28203230275514102, 4.000000000000006217 ) ) ;
#10590=DIRECTION ( 'NONE',  ( -1.000000000000000000, 8.326672684688672475E-15, 0.000000000000000000 ) ) ;
#10593=PLANE ( 'NONE',  #2157 ) ;
#10598=VECTOR ( 'NONE', #8856, 1000.000000000000000 ) ;
#10603=ORIENTED_EDGE ( 'NONE', *, *, #8776, .F. ) ;
#10635=CARTESIAN_POINT ( 'NONE',  ( -1.500000000000000444, 83.00000000000000000, -1.500000000000000222 ) ) ;
#10643=VECTOR ( 'NONE', #5513, 1000.000000000000000 ) ;
#10649=CARTESIAN_POINT ( 'NONE',  ( 67.97877056362573001, 94.28203230275514102, 5.000000000000000000 ) ) ;
#10652=LINE ( 'NONE', #5572, #1283 ) ;
#10674=FACE_OUTER_BOUND ( 'NONE', #9190, .T. ) ;
#10675=SURFACE_SIDE_STYLE ('',( #2108 ) ) ;
#10686=DIRECTION ( 'NONE',  ( -0.000000000000000000, -0.000000000000000000, 1.000000000000000000 ) ) ;
#10698=DIRECTION ( 'NONE',  ( 0.000000000000000000, 1.000000000000000000, 0.000000000000000000 ) ) ;
#10702=CARTESIAN_POINT ( 'NONE',  ( -10.00000000000000000, 90.00000000000001421, 5.000000000000000000 ) ) ;
#10713=EDGE_CURVE ( 'NONE', #1976, #564, #5773, .T. ) ;
#10714=ORIENTED_EDGE ( 'NONE', *, *, #3323, .T. ) ;
#10720=ORIENTED_EDGE ( 'NONE', *, *, #1610, .T. ) ;
#10725=CYLINDRICAL_SURFACE ( 'NONE', #5347, 4.999999999999987566 ) ;
#10726=DIRECTION ( 'NONE',  ( -0.000000000000000000, -0.000000000000000000, 1.000000000000000000 ) ) ;
#10730=ORIENTED_EDGE ( 'NONE', *, *, #4118, .T. ) ;
#10731=ORIENTED_EDGE ( 'NONE', *, *, #7663, .F. ) ;
#10756=PLANE ( 'NONE',  #8250 ) ;
#10757=CARTESIAN_POINT ( 'NONE',  ( 7.856406460551036197, 93.00000000000001421, -5.000000000000000000 ) ) ;
#10770=EDGE_CURVE ( 'NONE', #5226, #8103, #672, .T. ) ;
#10785=CARTESIAN_POINT ( 'NONE',  ( 67.32050807568876394, 92.28203230275514102, -5.000000000000000000 ) ) ;
#10794=AXIS2_PLACEMENT_3D ( 'NONE', #3189, #3997, #2478 ) ;
#10799=VECTOR ( 'NONE', #3001, 1000.000000000000000 ) ;
#10816=AXIS2_PLACEMENT_3D ( 'NONE', #7864, #4510, #7802 ) ;
#10820=AXIS2_PLACEMENT_3D ( 'NONE', #5778, #754, #7542 ) ;
#10828=AXIS2_PLACEMENT_3D ( 'NONE', #4033, #8173, #2204 ) ;
#10830=ORIENTED_EDGE ( 'NONE', *, *, #7732, .T. ) ;
#10838=DIRECTION ( 'NONE',  ( -1.000000000000000000, 0.000000000000000000, 1.445602896647339163E-16 ) ) ;
#10864=VERTEX_POINT ( 'NONE', #3307 ) ;
#10866=ORIENTED_EDGE ( 'NONE', *, *, #2267, .T. ) ;
#10879=ORIENTED_EDGE ( 'NONE', *, *, #377, .F. ) ;
#10880=DIRECTION ( 'NONE',  ( -1.000000000000000000, 0.000000000000000000, 0.000000000000000000 ) ) ;
#10891=CARTESIAN_POINT ( 'NONE',  ( 7.856406460551036197, 98.00000000000001421, 5.000000000000000000 ) ) ;
#10920=ADVANCED_FACE ( 'NONE', ( #2765 ), #5448, .T. ) ;
#10930=DIRECTION ( 'NONE',  ( 1.000000000000000000, 0.000000000000000000, 0.000000000000000000 ) ) ;
#10936=ADVANCED_FACE ( 'NONE', ( #973 ), #8961, .T. ) ;
#10938=ORIENTED_EDGE ( 'NONE', *, *, #5408, .T. ) ;
ENDSEC;
END-ISO-10303-21;
